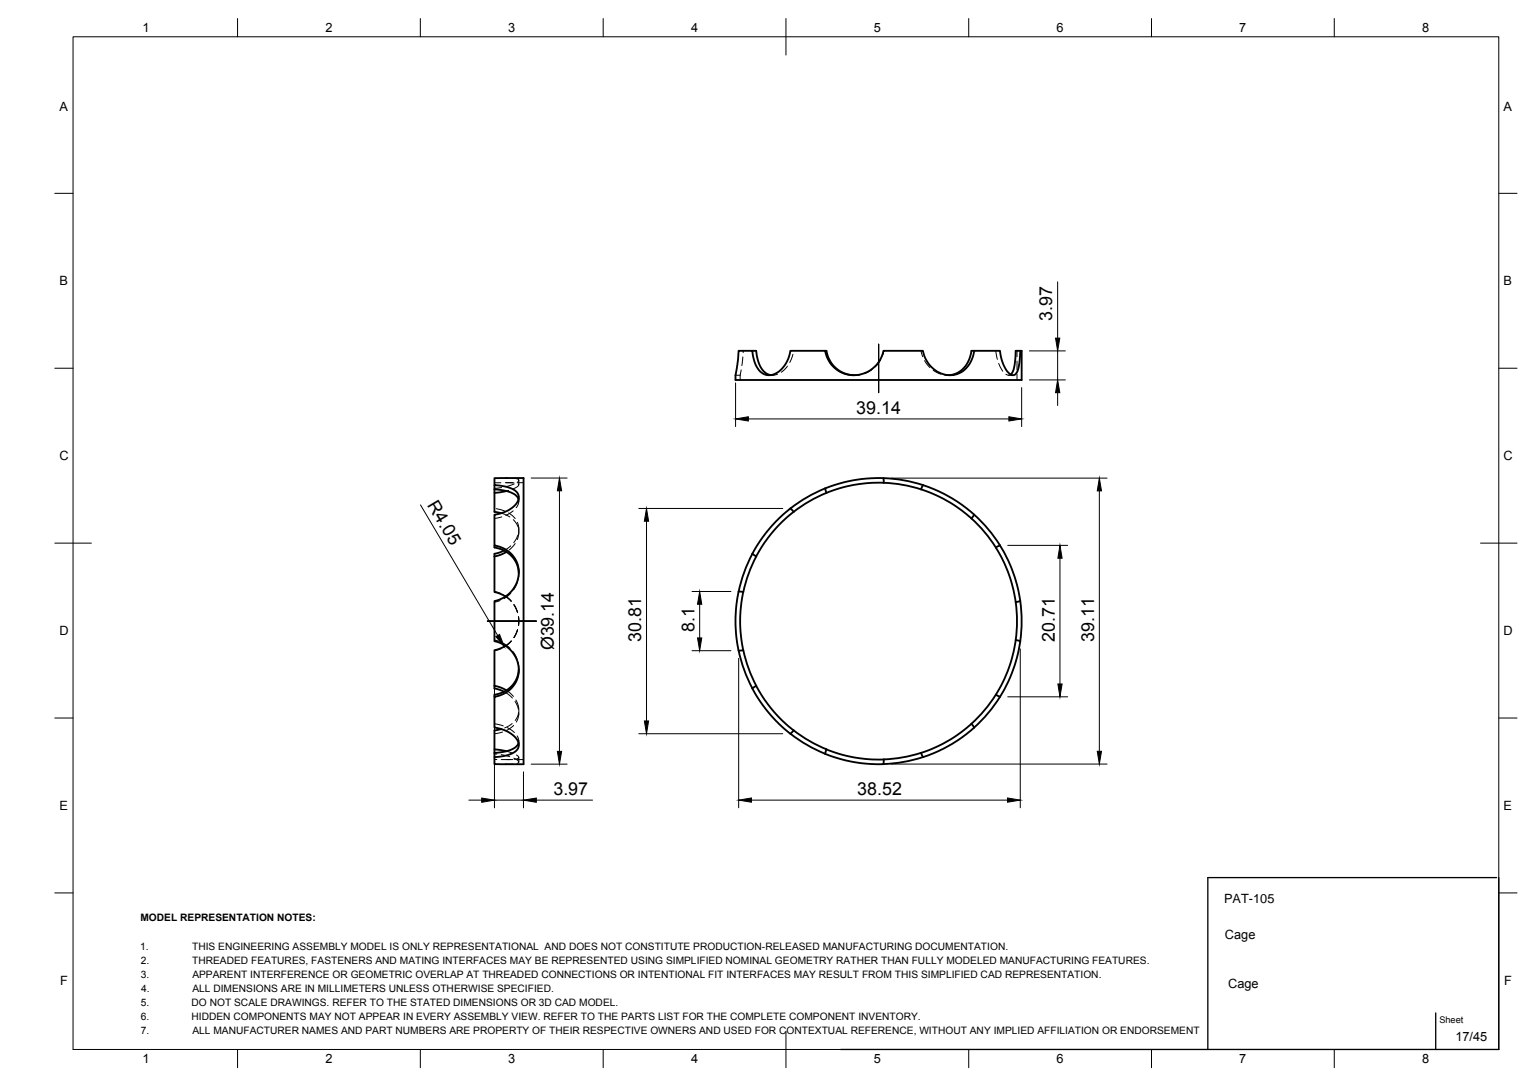
ISO-10303-21;
HEADER;
/* Generated by software containing ST-Developer
 * from STEP Tools, Inc. (www.steptools.com) 
 */

FILE_DESCRIPTION(
/* description */ ('Torque wrench calibration arm'),
/* implementation_level */ '2;1');

FILE_NAME(
/* name */ 'Cage.step',
/* time_stamp */ '2026-10-28T03:24:52-07:00',
/* author */ (''),
/* organization */ (''),
/* preprocessor_version */ 'ST-DEVELOPER v20.2',
/* originating_system */ 'Autodesk Translation Framework v15.17.0.0',
/* authorisation */ '');

FILE_SCHEMA (('AUTOMOTIVE_DESIGN { 1 0 10303 214 3 1 1 }'));
ENDSEC;

DATA;
#10=MECHANICAL_DESIGN_GEOMETRIC_PRESENTATION_REPRESENTATION('',(#444),#12783);
#245=B_SPLINE_CURVE_WITH_KNOTS('',3,(#10516,#10517,#10518,#10519,#10520,
#10521,#10522,#10523,#10524,#10525,#10526,#10527,#10528,#10529,#10530,#10531,
#10532,#10533,#10534,#10535,#10536,#10537),.UNSPECIFIED.,.F.,.F.,(4,2,2,
2,2,2,2,2,2,2,4),(0.0789043916784349,0.21052649634152,0.31578974451228,
0.421052992683041,0.522171766675512,0.623290540667983,0.724409314660453,
0.825528088652924,0.930791336823684,1.03605458499444,1.16767668965753),
 .UNSPECIFIED.);
#246=B_SPLINE_CURVE_WITH_KNOTS('',3,(#10541,#10542,#10543,#10544,#10545,
#10546,#10547,#10548,#10549,#10550,#10551,#10552,#10553,#10554,#10555,#10556,
#10557,#10558,#10559,#10560,#10561,#10562),.UNSPECIFIED.,.F.,.F.,(4,2,2,
2,2,2,2,2,2,2,4),(0.0774711646211702,0.142095081356994,0.284190162713987,
0.410912155766437,0.514012992401139,0.617113829035841,0.720214665670543,
0.823315502305246,0.950037495357694,1.09213257671469,1.15675649345051),
 .UNSPECIFIED.);
#247=B_SPLINE_CURVE_WITH_KNOTS('',3,(#10568,#10569,#10570,#10571,#10572,
#10573,#10574,#10575,#10576,#10577,#10578,#10579,#10580,#10581,#10582,#10583,
#10584,#10585,#10586,#10587,#10588,#10589),.UNSPECIFIED.,.F.,.F.,(4,2,2,
2,2,2,2,2,2,2,4),(0.0774711646211703,0.142095081356994,0.284190162713988,
0.410912155766436,0.514012992401139,0.617113829035841,0.720214665670544,
0.823315502305246,0.950037495357695,1.09213257671469,1.15675649345051),
 .UNSPECIFIED.);
#248=B_SPLINE_CURVE_WITH_KNOTS('',3,(#10593,#10594,#10595,#10596,#10597,
#10598,#10599,#10600,#10601,#10602,#10603,#10604,#10605,#10606,#10607,#10608,
#10609,#10610,#10611,#10612,#10613,#10614),.UNSPECIFIED.,.F.,.F.,(4,2,2,
2,2,2,2,2,2,2,4),(0.0774711646211702,0.142095081356994,0.284190162713988,
0.410912155766436,0.514012992401139,0.617113829035841,0.720214665670544,
0.823315502305246,0.950037495357695,1.09213257671469,1.15675649345051),
 .UNSPECIFIED.);
#249=B_SPLINE_CURVE_WITH_KNOTS('',3,(#10618,#10619,#10620,#10621,#10622,
#10623,#10624,#10625,#10626,#10627,#10628,#10629,#10630,#10631,#10632,#10633,
#10634,#10635,#10636,#10637,#10638,#10639),.UNSPECIFIED.,.F.,.F.,(4,2,2,
2,2,2,2,2,2,2,4),(0.0774711646211702,0.142095081356994,0.284190162713988,
0.410912155766436,0.514012992401139,0.617113829035842,0.720214665670544,
0.823315502305246,0.950037495357696,1.09213257671469,1.15675649345051),
 .UNSPECIFIED.);
#250=B_SPLINE_CURVE_WITH_KNOTS('',3,(#10648,#10649,#10650,#10651,#10652,
#10653,#10654,#10655,#10656,#10657,#10658,#10659,#10660,#10661,#10662,#10663,
#10664,#10665,#10666,#10667,#10668,#10669),.UNSPECIFIED.,.F.,.F.,(4,2,2,
2,2,2,2,2,2,2,4),(0.0774711646211702,0.142095081356994,0.284190162713987,
0.410912155766436,0.514012992401139,0.617113829035841,0.720214665670543,
0.823315502305246,0.950037495357695,1.09213257671469,1.15675649345051),
 .UNSPECIFIED.);
#251=B_SPLINE_CURVE_WITH_KNOTS('',3,(#10673,#10674,#10675,#10676,#10677,
#10678,#10679,#10680,#10681,#10682,#10683,#10684,#10685,#10686,#10687,#10688,
#10689,#10690,#10691,#10692,#10693,#10694),.UNSPECIFIED.,.F.,.F.,(4,2,2,
2,2,2,2,2,2,2,4),(0.0774711646211702,0.142095081356994,0.284190162713987,
0.410912155766436,0.514012992401139,0.617113829035841,0.720214665670543,
0.823315502305246,0.950037495357695,1.09213257671469,1.15675649345051),
 .UNSPECIFIED.);
#252=B_SPLINE_CURVE_WITH_KNOTS('',3,(#10698,#10699,#10700,#10701,#10702,
#10703,#10704,#10705,#10706,#10707,#10708,#10709,#10710,#10711,#10712,#10713,
#10714,#10715,#10716,#10717,#10718,#10719),.UNSPECIFIED.,.F.,.F.,(4,2,2,
2,2,2,2,2,2,2,4),(0.0774711646211703,0.142095081356994,0.284190162713988,
0.410912155766437,0.514012992401139,0.617113829035841,0.720214665670544,
0.823315502305247,0.950037495357696,1.09213257671469,1.15675649345051),
 .UNSPECIFIED.);
#253=B_SPLINE_CURVE_WITH_KNOTS('',3,(#10723,#10724,#10725,#10726,#10727,
#10728,#10729,#10730,#10731,#10732,#10733,#10734,#10735,#10736,#10737,#10738,
#10739,#10740,#10741,#10742,#10743,#10744),.UNSPECIFIED.,.F.,.F.,(4,2,2,
2,2,2,2,2,2,2,4),(0.0774711646211703,0.142095081356994,0.284190162713987,
0.410912155766436,0.514012992401139,0.617113829035841,0.720214665670543,
0.823315502305245,0.950037495357694,1.09213257671469,1.15675649345051),
 .UNSPECIFIED.);
#254=B_SPLINE_CURVE_WITH_KNOTS('',3,(#10748,#10749,#10750,#10751,#10752,
#10753,#10754,#10755,#10756,#10757,#10758,#10759,#10760,#10761,#10762,#10763,
#10764,#10765,#10766,#10767,#10768,#10769),.UNSPECIFIED.,.F.,.F.,(4,2,2,
2,2,2,2,2,2,2,4),(0.0774711646211703,0.142095081356994,0.284190162713988,
0.410912155766437,0.514012992401139,0.617113829035841,0.720214665670544,
0.823315502305246,0.950037495357695,1.09213257671469,1.15675649345051),
 .UNSPECIFIED.);
#255=B_SPLINE_CURVE_WITH_KNOTS('',3,(#10777,#10778,#10779,#10780,#10781,
#10782,#10783,#10784,#10785,#10786,#10787,#10788,#10789,#10790,#10791,#10792,
#10793,#10794,#10795,#10796,#10797,#10798),.UNSPECIFIED.,.F.,.F.,(4,2,2,
2,2,2,2,2,2,2,4),(0.0789043916784349,0.21052649634152,0.315789744512281,
0.421052992683041,0.522171766675512,0.623290540667983,0.724409314660453,
0.825528088652924,0.930791336823684,1.03605458499444,1.16767668965753),
 .UNSPECIFIED.);
#256=B_SPLINE_CURVE_WITH_KNOTS('',3,(#10806,#10807,#10808,#10809,#10810,
#10811,#10812,#10813,#10814,#10815,#10816,#10817,#10818,#10819,#10820,#10821,
#10822,#10823,#10824,#10825,#10826,#10827),.UNSPECIFIED.,.F.,.F.,(4,2,2,
2,2,2,2,2,2,2,4),(0.0789043916784348,0.210526496341521,0.315789744512281,
0.421052992683042,0.522171766675513,0.623290540667983,0.724409314660454,
0.825528088652925,0.930791336823685,1.03605458499444,1.16767668965753),
 .UNSPECIFIED.);
#257=B_SPLINE_CURVE_WITH_KNOTS('',3,(#10835,#10836,#10837,#10838,#10839,
#10840,#10841,#10842,#10843,#10844,#10845,#10846,#10847,#10848,#10849,#10850,
#10851,#10852,#10853,#10854,#10855,#10856),.UNSPECIFIED.,.F.,.F.,(4,2,2,
2,2,2,2,2,2,2,4),(0.0789043916784349,0.21052649634152,0.31578974451228,
0.421052992683041,0.522171766675511,0.623290540667982,0.724409314660453,
0.825528088652924,0.930791336823685,1.03605458499444,1.16767668965753),
 .UNSPECIFIED.);
#258=B_SPLINE_CURVE_WITH_KNOTS('',3,(#10866,#10867,#10868,#10869,#10870,
#10871,#10872,#10873,#10874,#10875,#10876,#10877,#10878,#10879,#10880,#10881,
#10882,#10883,#10884,#10885,#10886,#10887),.UNSPECIFIED.,.F.,.F.,(4,2,2,
2,2,2,2,2,2,2,4),(0.0789043916784348,0.21052649634152,0.315789744512281,
0.421052992683041,0.522171766675511,0.623290540667982,0.724409314660453,
0.825528088652924,0.930791336823684,1.03605458499444,1.16767668965753),
 .UNSPECIFIED.);
#259=B_SPLINE_CURVE_WITH_KNOTS('',3,(#10895,#10896,#10897,#10898,#10899,
#10900,#10901,#10902,#10903,#10904,#10905,#10906,#10907,#10908,#10909,#10910,
#10911,#10912,#10913,#10914,#10915,#10916),.UNSPECIFIED.,.F.,.F.,(4,2,2,
2,2,2,2,2,2,2,4),(0.0789043916784348,0.21052649634152,0.31578974451228,
0.42105299268304,0.522171766675511,0.623290540667982,0.724409314660453,
0.825528088652924,0.930791336823684,1.03605458499444,1.16767668965753),
 .UNSPECIFIED.);
#260=B_SPLINE_CURVE_WITH_KNOTS('',3,(#10924,#10925,#10926,#10927,#10928,
#10929,#10930,#10931,#10932,#10933,#10934,#10935,#10936,#10937,#10938,#10939,
#10940,#10941,#10942,#10943,#10944,#10945),.UNSPECIFIED.,.F.,.F.,(4,2,2,
2,2,2,2,2,2,2,4),(0.0789043916784348,0.21052649634152,0.315789744512281,
0.421052992683041,0.522171766675512,0.623290540667982,0.724409314660453,
0.825528088652924,0.930791336823684,1.03605458499444,1.16767668965753),
 .UNSPECIFIED.);
#261=B_SPLINE_CURVE_WITH_KNOTS('',3,(#10953,#10954,#10955,#10956,#10957,
#10958,#10959,#10960,#10961,#10962,#10963,#10964,#10965,#10966,#10967,#10968,
#10969,#10970,#10971,#10972,#10973,#10974),.UNSPECIFIED.,.F.,.F.,(4,2,2,
2,2,2,2,2,2,2,4),(0.0789043916784349,0.21052649634152,0.31578974451228,
0.42105299268304,0.522171766675511,0.623290540667982,0.724409314660453,
0.825528088652924,0.930791336823684,1.03605458499444,1.16767668965753),
 .UNSPECIFIED.);
#262=B_SPLINE_CURVE_WITH_KNOTS('',3,(#10983,#10984,#10985,#10986,#10987,
#10988,#10989,#10990,#10991,#10992,#10993,#10994,#10995,#10996,#10997,#10998,
#10999,#11000,#11001,#11002,#11003,#11004),.UNSPECIFIED.,.F.,.F.,(4,2,2,
2,2,2,2,2,2,2,4),(0.0789043916784348,0.21052649634152,0.31578974451228,
0.42105299268304,0.522171766675511,0.623290540667982,0.724409314660453,
0.825528088652924,0.930791336823684,1.03605458499444,1.16767668965753),
 .UNSPECIFIED.);
#302=SPHERICAL_SURFACE('',#7218,0.412776);
#303=SPHERICAL_SURFACE('',#7236,0.412776);
#304=SPHERICAL_SURFACE('',#7241,0.412776);
#305=SPHERICAL_SURFACE('',#7246,0.412776);
#306=SPHERICAL_SURFACE('',#7252,0.412776);
#307=SPHERICAL_SURFACE('',#7257,0.412776);
#308=SPHERICAL_SURFACE('',#7262,0.412776);
#309=SPHERICAL_SURFACE('',#7267,0.412776);
#310=SPHERICAL_SURFACE('',#7275,0.412776);
#362=SHAPE_REPRESENTATION_RELATIONSHIP('SRR','None',#12944,#399);
#399=ADVANCED_BREP_SHAPE_REPRESENTATION('',(#498),#12753);
#444=STYLED_ITEM('',(#13212),#498);
#498=MANIFOLD_SOLID_BREP('Continuous crown cage',#6513);
#587=FACE_BOUND('',#1471,.T.);
#714=PLANE('',#7233);
#715=PLANE('',#7238);
#716=PLANE('',#7243);
#717=PLANE('',#7248);
#718=PLANE('',#7254);
#719=PLANE('',#7259);
#720=PLANE('',#7264);
#721=PLANE('',#7273);
#722=PLANE('',#7277);
#723=PLANE('',#7278);
#1000=FACE_OUTER_BOUND('',#1451,.T.);
#1001=FACE_OUTER_BOUND('',#1452,.T.);
#1002=FACE_OUTER_BOUND('',#1453,.T.);
#1003=FACE_OUTER_BOUND('',#1454,.T.);
#1004=FACE_OUTER_BOUND('',#1455,.T.);
#1005=FACE_OUTER_BOUND('',#1456,.T.);
#1006=FACE_OUTER_BOUND('',#1457,.T.);
#1007=FACE_OUTER_BOUND('',#1458,.T.);
#1008=FACE_OUTER_BOUND('',#1459,.T.);
#1009=FACE_OUTER_BOUND('',#1460,.T.);
#1010=FACE_OUTER_BOUND('',#1461,.T.);
#1011=FACE_OUTER_BOUND('',#1462,.T.);
#1012=FACE_OUTER_BOUND('',#1463,.T.);
#1013=FACE_OUTER_BOUND('',#1464,.T.);
#1014=FACE_OUTER_BOUND('',#1465,.T.);
#1015=FACE_OUTER_BOUND('',#1466,.T.);
#1016=FACE_OUTER_BOUND('',#1467,.T.);
#1017=FACE_OUTER_BOUND('',#1468,.T.);
#1018=FACE_OUTER_BOUND('',#1469,.T.);
#1019=FACE_OUTER_BOUND('',#1470,.T.);
#1020=FACE_OUTER_BOUND('',#1472,.T.);
#1451=EDGE_LOOP('',(#4877,#4878,#4879,#4880));
#1452=EDGE_LOOP('',(#4881,#4882,#4883,#4884,#4885,#4886,#4887,#4888,#4889,
#4890,#4891,#4892,#4893,#4894,#4895,#4896,#4897,#4898,#4899,#4900,#4901,
#4902));
#1453=EDGE_LOOP('',(#4903,#4904,#4905,#4906));
#1454=EDGE_LOOP('',(#4907,#4908,#4909,#4910));
#1455=EDGE_LOOP('',(#4911,#4912,#4913,#4914));
#1456=EDGE_LOOP('',(#4915,#4916,#4917,#4918));
#1457=EDGE_LOOP('',(#4919,#4920,#4921,#4922));
#1458=EDGE_LOOP('',(#4923,#4924,#4925,#4926));
#1459=EDGE_LOOP('',(#4927,#4928,#4929,#4930,#4931,#4932));
#1460=EDGE_LOOP('',(#4933,#4934,#4935,#4936));
#1461=EDGE_LOOP('',(#4937,#4938,#4939,#4940));
#1462=EDGE_LOOP('',(#4941,#4942,#4943,#4944));
#1463=EDGE_LOOP('',(#4945,#4946,#4947,#4948));
#1464=EDGE_LOOP('',(#4949,#4950,#4951,#4952));
#1465=EDGE_LOOP('',(#4953,#4954,#4955,#4956));
#1466=EDGE_LOOP('',(#4957,#4958,#4959,#4960));
#1467=EDGE_LOOP('',(#4961,#4962,#4963,#4964,#4965,#4966,#4967,#4968,#4969,
#4970,#4971,#4972,#4973,#4974,#4975,#4976,#4977,#4978,#4979,#4980,#4981,
#4982));
#1468=EDGE_LOOP('',(#4983,#4984,#4985,#4986));
#1469=EDGE_LOOP('',(#4987,#4988,#4989,#4990));
#1470=EDGE_LOOP('',(#4991));
#1471=EDGE_LOOP('',(#4992));
#1472=EDGE_LOOP('',(#4993,#4994,#4995,#4996));
#1930=LINE('',#10643,#2345);
#1931=LINE('',#10979,#2346);
#2345=VECTOR('',#8486,1.956752);
#2346=VECTOR('',#8577,1.893248);
#2735=CIRCLE('',#7219,0.405071403305639);
#2736=CIRCLE('',#7220,0.405071403305639);
#2737=CIRCLE('',#7222,1.956752);
#2738=CIRCLE('',#7223,1.956752);
#2739=CIRCLE('',#7224,1.956752);
#2740=CIRCLE('',#7225,1.956752);
#2741=CIRCLE('',#7226,1.956752);
#2742=CIRCLE('',#7227,1.956752);
#2743=CIRCLE('',#7228,1.956752);
#2744=CIRCLE('',#7229,1.956752);
#2745=CIRCLE('',#7230,1.956752);
#2746=CIRCLE('',#7231,1.956752);
#2747=CIRCLE('',#7232,1.956752);
#2748=CIRCLE('',#7234,1.893248);
#2749=CIRCLE('',#7235,0.405071403305639);
#2750=CIRCLE('',#7237,0.405071403305639);
#2751=CIRCLE('',#7239,1.893248);
#2752=CIRCLE('',#7240,0.405071403305639);
#2753=CIRCLE('',#7242,0.405071403305639);
#2754=CIRCLE('',#7244,1.893248);
#2755=CIRCLE('',#7245,0.405071403305639);
#2756=CIRCLE('',#7247,0.405071403305639);
#2757=CIRCLE('',#7249,1.893248);
#2758=CIRCLE('',#7250,1.893248);
#2759=CIRCLE('',#7251,0.405071403305639);
#2760=CIRCLE('',#7253,0.405071403305639);
#2761=CIRCLE('',#7255,1.893248);
#2762=CIRCLE('',#7256,0.405071403305639);
#2763=CIRCLE('',#7258,0.405071403305639);
#2764=CIRCLE('',#7260,1.893248);
#2765=CIRCLE('',#7261,0.405071403305639);
#2766=CIRCLE('',#7263,0.405071403305639);
#2767=CIRCLE('',#7265,1.893248);
#2768=CIRCLE('',#7266,0.405071403305639);
#2769=CIRCLE('',#7268,0.405071403305639);
#2770=CIRCLE('',#7270,1.893248);
#2771=CIRCLE('',#7271,1.893248);
#2772=CIRCLE('',#7272,1.893248);
#2773=CIRCLE('',#7274,0.405071403305639);
#2774=CIRCLE('',#7276,0.405071403305639);
#3157=VERTEX_POINT('',#10514);
#3158=VERTEX_POINT('',#10515);
#3159=VERTEX_POINT('',#10538);
#3160=VERTEX_POINT('',#10540);
#3161=VERTEX_POINT('',#10565);
#3162=VERTEX_POINT('',#10567);
#3163=VERTEX_POINT('',#10590);
#3164=VERTEX_POINT('',#10592);
#3165=VERTEX_POINT('',#10615);
#3166=VERTEX_POINT('',#10617);
#3167=VERTEX_POINT('',#10640);
#3168=VERTEX_POINT('',#10642);
#3169=VERTEX_POINT('',#10645);
#3170=VERTEX_POINT('',#10647);
#3171=VERTEX_POINT('',#10670);
#3172=VERTEX_POINT('',#10672);
#3173=VERTEX_POINT('',#10695);
#3174=VERTEX_POINT('',#10697);
#3175=VERTEX_POINT('',#10720);
#3176=VERTEX_POINT('',#10722);
#3177=VERTEX_POINT('',#10745);
#3178=VERTEX_POINT('',#10747);
#3179=VERTEX_POINT('',#10772);
#3180=VERTEX_POINT('',#10776);
#3181=VERTEX_POINT('',#10801);
#3182=VERTEX_POINT('',#10805);
#3183=VERTEX_POINT('',#10830);
#3184=VERTEX_POINT('',#10834);
#3185=VERTEX_POINT('',#10859);
#3186=VERTEX_POINT('',#10861);
#3187=VERTEX_POINT('',#10865);
#3188=VERTEX_POINT('',#10890);
#3189=VERTEX_POINT('',#10894);
#3190=VERTEX_POINT('',#10919);
#3191=VERTEX_POINT('',#10923);
#3192=VERTEX_POINT('',#10948);
#3193=VERTEX_POINT('',#10952);
#3194=VERTEX_POINT('',#10977);
#3195=VERTEX_POINT('',#10980);
#3196=VERTEX_POINT('',#10982);
#3796=EDGE_CURVE('',#3157,#3158,#245,.T.);
#3797=EDGE_CURVE('',#3159,#3157,#2735,.T.);
#3798=EDGE_CURVE('',#3160,#3159,#246,.T.);
#3799=EDGE_CURVE('',#3158,#3160,#2736,.T.);
#3800=EDGE_CURVE('',#3161,#3159,#2737,.T.);
#3801=EDGE_CURVE('',#3161,#3162,#247,.T.);
#3802=EDGE_CURVE('',#3163,#3162,#2738,.T.);
#3803=EDGE_CURVE('',#3163,#3164,#248,.T.);
#3804=EDGE_CURVE('',#3165,#3164,#2739,.T.);
#3805=EDGE_CURVE('',#3165,#3166,#249,.T.);
#3806=EDGE_CURVE('',#3167,#3166,#2740,.T.);
#3807=EDGE_CURVE('',#3167,#3168,#1930,.T.);
#3808=EDGE_CURVE('',#3168,#3168,#2741,.T.);
#3809=EDGE_CURVE('',#3169,#3167,#2742,.T.);
#3810=EDGE_CURVE('',#3169,#3170,#250,.T.);
#3811=EDGE_CURVE('',#3171,#3170,#2743,.T.);
#3812=EDGE_CURVE('',#3171,#3172,#251,.T.);
#3813=EDGE_CURVE('',#3173,#3172,#2744,.T.);
#3814=EDGE_CURVE('',#3173,#3174,#252,.T.);
#3815=EDGE_CURVE('',#3175,#3174,#2745,.T.);
#3816=EDGE_CURVE('',#3175,#3176,#253,.T.);
#3817=EDGE_CURVE('',#3177,#3176,#2746,.T.);
#3818=EDGE_CURVE('',#3177,#3178,#254,.T.);
#3819=EDGE_CURVE('',#3160,#3178,#2747,.T.);
#3820=EDGE_CURVE('',#3157,#3179,#2748,.T.);
#3821=EDGE_CURVE('',#3179,#3161,#2749,.T.);
#3822=EDGE_CURVE('',#3180,#3179,#255,.T.);
#3823=EDGE_CURVE('',#3162,#3180,#2750,.T.);
#3824=EDGE_CURVE('',#3180,#3181,#2751,.T.);
#3825=EDGE_CURVE('',#3181,#3163,#2752,.T.);
#3826=EDGE_CURVE('',#3182,#3181,#256,.T.);
#3827=EDGE_CURVE('',#3164,#3182,#2753,.T.);
#3828=EDGE_CURVE('',#3182,#3183,#2754,.T.);
#3829=EDGE_CURVE('',#3183,#3165,#2755,.T.);
#3830=EDGE_CURVE('',#3184,#3183,#257,.T.);
#3831=EDGE_CURVE('',#3166,#3184,#2756,.T.);
#3832=EDGE_CURVE('',#3184,#3185,#2757,.T.);
#3833=EDGE_CURVE('',#3185,#3186,#2758,.T.);
#3834=EDGE_CURVE('',#3186,#3169,#2759,.T.);
#3835=EDGE_CURVE('',#3187,#3186,#258,.T.);
#3836=EDGE_CURVE('',#3170,#3187,#2760,.T.);
#3837=EDGE_CURVE('',#3187,#3188,#2761,.T.);
#3838=EDGE_CURVE('',#3188,#3171,#2762,.T.);
#3839=EDGE_CURVE('',#3189,#3188,#259,.T.);
#3840=EDGE_CURVE('',#3172,#3189,#2763,.T.);
#3841=EDGE_CURVE('',#3189,#3190,#2764,.T.);
#3842=EDGE_CURVE('',#3190,#3173,#2765,.T.);
#3843=EDGE_CURVE('',#3191,#3190,#260,.T.);
#3844=EDGE_CURVE('',#3174,#3191,#2766,.T.);
#3845=EDGE_CURVE('',#3191,#3192,#2767,.T.);
#3846=EDGE_CURVE('',#3192,#3175,#2768,.T.);
#3847=EDGE_CURVE('',#3193,#3192,#261,.T.);
#3848=EDGE_CURVE('',#3176,#3193,#2769,.T.);
#3849=EDGE_CURVE('',#3194,#3194,#2770,.T.);
#3850=EDGE_CURVE('',#3194,#3185,#1931,.T.);
#3851=EDGE_CURVE('',#3195,#3158,#2771,.T.);
#3852=EDGE_CURVE('',#3195,#3196,#262,.T.);
#3853=EDGE_CURVE('',#3193,#3196,#2772,.T.);
#3854=EDGE_CURVE('',#3178,#3195,#2773,.T.);
#3855=EDGE_CURVE('',#3196,#3177,#2774,.T.);
#4877=ORIENTED_EDGE('',*,*,#3796,.F.);
#4878=ORIENTED_EDGE('',*,*,#3797,.F.);
#4879=ORIENTED_EDGE('',*,*,#3798,.F.);
#4880=ORIENTED_EDGE('',*,*,#3799,.F.);
#4881=ORIENTED_EDGE('',*,*,#3798,.T.);
#4882=ORIENTED_EDGE('',*,*,#3800,.F.);
#4883=ORIENTED_EDGE('',*,*,#3801,.T.);
#4884=ORIENTED_EDGE('',*,*,#3802,.F.);
#4885=ORIENTED_EDGE('',*,*,#3803,.T.);
#4886=ORIENTED_EDGE('',*,*,#3804,.F.);
#4887=ORIENTED_EDGE('',*,*,#3805,.T.);
#4888=ORIENTED_EDGE('',*,*,#3806,.F.);
#4889=ORIENTED_EDGE('',*,*,#3807,.T.);
#4890=ORIENTED_EDGE('',*,*,#3808,.F.);
#4891=ORIENTED_EDGE('',*,*,#3807,.F.);
#4892=ORIENTED_EDGE('',*,*,#3809,.F.);
#4893=ORIENTED_EDGE('',*,*,#3810,.T.);
#4894=ORIENTED_EDGE('',*,*,#3811,.F.);
#4895=ORIENTED_EDGE('',*,*,#3812,.T.);
#4896=ORIENTED_EDGE('',*,*,#3813,.F.);
#4897=ORIENTED_EDGE('',*,*,#3814,.T.);
#4898=ORIENTED_EDGE('',*,*,#3815,.F.);
#4899=ORIENTED_EDGE('',*,*,#3816,.T.);
#4900=ORIENTED_EDGE('',*,*,#3817,.F.);
#4901=ORIENTED_EDGE('',*,*,#3818,.T.);
#4902=ORIENTED_EDGE('',*,*,#3819,.F.);
#4903=ORIENTED_EDGE('',*,*,#3797,.T.);
#4904=ORIENTED_EDGE('',*,*,#3820,.T.);
#4905=ORIENTED_EDGE('',*,*,#3821,.T.);
#4906=ORIENTED_EDGE('',*,*,#3800,.T.);
#4907=ORIENTED_EDGE('',*,*,#3822,.F.);
#4908=ORIENTED_EDGE('',*,*,#3823,.F.);
#4909=ORIENTED_EDGE('',*,*,#3801,.F.);
#4910=ORIENTED_EDGE('',*,*,#3821,.F.);
#4911=ORIENTED_EDGE('',*,*,#3823,.T.);
#4912=ORIENTED_EDGE('',*,*,#3824,.T.);
#4913=ORIENTED_EDGE('',*,*,#3825,.T.);
#4914=ORIENTED_EDGE('',*,*,#3802,.T.);
#4915=ORIENTED_EDGE('',*,*,#3826,.F.);
#4916=ORIENTED_EDGE('',*,*,#3827,.F.);
#4917=ORIENTED_EDGE('',*,*,#3803,.F.);
#4918=ORIENTED_EDGE('',*,*,#3825,.F.);
#4919=ORIENTED_EDGE('',*,*,#3827,.T.);
#4920=ORIENTED_EDGE('',*,*,#3828,.T.);
#4921=ORIENTED_EDGE('',*,*,#3829,.T.);
#4922=ORIENTED_EDGE('',*,*,#3804,.T.);
#4923=ORIENTED_EDGE('',*,*,#3830,.F.);
#4924=ORIENTED_EDGE('',*,*,#3831,.F.);
#4925=ORIENTED_EDGE('',*,*,#3805,.F.);
#4926=ORIENTED_EDGE('',*,*,#3829,.F.);
#4927=ORIENTED_EDGE('',*,*,#3831,.T.);
#4928=ORIENTED_EDGE('',*,*,#3832,.T.);
#4929=ORIENTED_EDGE('',*,*,#3833,.T.);
#4930=ORIENTED_EDGE('',*,*,#3834,.T.);
#4931=ORIENTED_EDGE('',*,*,#3809,.T.);
#4932=ORIENTED_EDGE('',*,*,#3806,.T.);
#4933=ORIENTED_EDGE('',*,*,#3835,.F.);
#4934=ORIENTED_EDGE('',*,*,#3836,.F.);
#4935=ORIENTED_EDGE('',*,*,#3810,.F.);
#4936=ORIENTED_EDGE('',*,*,#3834,.F.);
#4937=ORIENTED_EDGE('',*,*,#3836,.T.);
#4938=ORIENTED_EDGE('',*,*,#3837,.T.);
#4939=ORIENTED_EDGE('',*,*,#3838,.T.);
#4940=ORIENTED_EDGE('',*,*,#3811,.T.);
#4941=ORIENTED_EDGE('',*,*,#3839,.F.);
#4942=ORIENTED_EDGE('',*,*,#3840,.F.);
#4943=ORIENTED_EDGE('',*,*,#3812,.F.);
#4944=ORIENTED_EDGE('',*,*,#3838,.F.);
#4945=ORIENTED_EDGE('',*,*,#3840,.T.);
#4946=ORIENTED_EDGE('',*,*,#3841,.T.);
#4947=ORIENTED_EDGE('',*,*,#3842,.T.);
#4948=ORIENTED_EDGE('',*,*,#3813,.T.);
#4949=ORIENTED_EDGE('',*,*,#3843,.F.);
#4950=ORIENTED_EDGE('',*,*,#3844,.F.);
#4951=ORIENTED_EDGE('',*,*,#3814,.F.);
#4952=ORIENTED_EDGE('',*,*,#3842,.F.);
#4953=ORIENTED_EDGE('',*,*,#3844,.T.);
#4954=ORIENTED_EDGE('',*,*,#3845,.T.);
#4955=ORIENTED_EDGE('',*,*,#3846,.T.);
#4956=ORIENTED_EDGE('',*,*,#3815,.T.);
#4957=ORIENTED_EDGE('',*,*,#3816,.F.);
#4958=ORIENTED_EDGE('',*,*,#3846,.F.);
#4959=ORIENTED_EDGE('',*,*,#3847,.F.);
#4960=ORIENTED_EDGE('',*,*,#3848,.F.);
#4961=ORIENTED_EDGE('',*,*,#3849,.F.);
#4962=ORIENTED_EDGE('',*,*,#3850,.T.);
#4963=ORIENTED_EDGE('',*,*,#3832,.F.);
#4964=ORIENTED_EDGE('',*,*,#3830,.T.);
#4965=ORIENTED_EDGE('',*,*,#3828,.F.);
#4966=ORIENTED_EDGE('',*,*,#3826,.T.);
#4967=ORIENTED_EDGE('',*,*,#3824,.F.);
#4968=ORIENTED_EDGE('',*,*,#3822,.T.);
#4969=ORIENTED_EDGE('',*,*,#3820,.F.);
#4970=ORIENTED_EDGE('',*,*,#3796,.T.);
#4971=ORIENTED_EDGE('',*,*,#3851,.F.);
#4972=ORIENTED_EDGE('',*,*,#3852,.T.);
#4973=ORIENTED_EDGE('',*,*,#3853,.F.);
#4974=ORIENTED_EDGE('',*,*,#3847,.T.);
#4975=ORIENTED_EDGE('',*,*,#3845,.F.);
#4976=ORIENTED_EDGE('',*,*,#3843,.T.);
#4977=ORIENTED_EDGE('',*,*,#3841,.F.);
#4978=ORIENTED_EDGE('',*,*,#3839,.T.);
#4979=ORIENTED_EDGE('',*,*,#3837,.F.);
#4980=ORIENTED_EDGE('',*,*,#3835,.T.);
#4981=ORIENTED_EDGE('',*,*,#3833,.F.);
#4982=ORIENTED_EDGE('',*,*,#3850,.F.);
#4983=ORIENTED_EDGE('',*,*,#3799,.T.);
#4984=ORIENTED_EDGE('',*,*,#3819,.T.);
#4985=ORIENTED_EDGE('',*,*,#3854,.T.);
#4986=ORIENTED_EDGE('',*,*,#3851,.T.);
#4987=ORIENTED_EDGE('',*,*,#3818,.F.);
#4988=ORIENTED_EDGE('',*,*,#3855,.F.);
#4989=ORIENTED_EDGE('',*,*,#3852,.F.);
#4990=ORIENTED_EDGE('',*,*,#3854,.F.);
#4991=ORIENTED_EDGE('',*,*,#3808,.T.);
#4992=ORIENTED_EDGE('',*,*,#3849,.T.);
#4993=ORIENTED_EDGE('',*,*,#3848,.T.);
#4994=ORIENTED_EDGE('',*,*,#3853,.T.);
#4995=ORIENTED_EDGE('',*,*,#3855,.T.);
#4996=ORIENTED_EDGE('',*,*,#3817,.T.);
#6035=CYLINDRICAL_SURFACE('',#7221,1.956752);
#6036=CYLINDRICAL_SURFACE('',#7269,1.893248);
#6225=ADVANCED_FACE('',(#1000),#302,.F.);
#6226=ADVANCED_FACE('',(#1001),#6035,.T.);
#6227=ADVANCED_FACE('',(#1002),#714,.T.);
#6228=ADVANCED_FACE('',(#1003),#303,.F.);
#6229=ADVANCED_FACE('',(#1004),#715,.T.);
#6230=ADVANCED_FACE('',(#1005),#304,.F.);
#6231=ADVANCED_FACE('',(#1006),#716,.T.);
#6232=ADVANCED_FACE('',(#1007),#305,.F.);
#6233=ADVANCED_FACE('',(#1008),#717,.T.);
#6234=ADVANCED_FACE('',(#1009),#306,.F.);
#6235=ADVANCED_FACE('',(#1010),#718,.T.);
#6236=ADVANCED_FACE('',(#1011),#307,.F.);
#6237=ADVANCED_FACE('',(#1012),#719,.T.);
#6238=ADVANCED_FACE('',(#1013),#308,.F.);
#6239=ADVANCED_FACE('',(#1014),#720,.T.);
#6240=ADVANCED_FACE('',(#1015),#309,.F.);
#6241=ADVANCED_FACE('',(#1016),#6036,.F.);
#6242=ADVANCED_FACE('',(#1017),#721,.T.);
#6243=ADVANCED_FACE('',(#1018),#310,.F.);
#6244=ADVANCED_FACE('',(#1019,#587),#722,.T.);
#6245=ADVANCED_FACE('',(#1020),#723,.T.);
#6513=CLOSED_SHELL('',(#6225,#6226,#6227,#6228,#6229,#6230,#6231,#6232,
#6233,#6234,#6235,#6236,#6237,#6238,#6239,#6240,#6241,#6242,#6243,#6244,
#6245));
#7217=AXIS2_PLACEMENT_3D('',#10512,#8468,#8469);
#7218=AXIS2_PLACEMENT_3D('',#10513,#8470,#8471);
#7219=AXIS2_PLACEMENT_3D('',#10539,#8472,#8473);
#7220=AXIS2_PLACEMENT_3D('',#10563,#8474,#8475);
#7221=AXIS2_PLACEMENT_3D('',#10564,#8476,#8477);
#7222=AXIS2_PLACEMENT_3D('',#10566,#8478,#8479);
#7223=AXIS2_PLACEMENT_3D('',#10591,#8480,#8481);
#7224=AXIS2_PLACEMENT_3D('',#10616,#8482,#8483);
#7225=AXIS2_PLACEMENT_3D('',#10641,#8484,#8485);
#7226=AXIS2_PLACEMENT_3D('',#10644,#8487,#8488);
#7227=AXIS2_PLACEMENT_3D('',#10646,#8489,#8490);
#7228=AXIS2_PLACEMENT_3D('',#10671,#8491,#8492);
#7229=AXIS2_PLACEMENT_3D('',#10696,#8493,#8494);
#7230=AXIS2_PLACEMENT_3D('',#10721,#8495,#8496);
#7231=AXIS2_PLACEMENT_3D('',#10746,#8497,#8498);
#7232=AXIS2_PLACEMENT_3D('',#10770,#8499,#8500);
#7233=AXIS2_PLACEMENT_3D('',#10771,#8501,#8502);
#7234=AXIS2_PLACEMENT_3D('',#10773,#8503,#8504);
#7235=AXIS2_PLACEMENT_3D('',#10774,#8505,#8506);
#7236=AXIS2_PLACEMENT_3D('',#10775,#8507,#8508);
#7237=AXIS2_PLACEMENT_3D('',#10799,#8509,#8510);
#7238=AXIS2_PLACEMENT_3D('',#10800,#8511,#8512);
#7239=AXIS2_PLACEMENT_3D('',#10802,#8513,#8514);
#7240=AXIS2_PLACEMENT_3D('',#10803,#8515,#8516);
#7241=AXIS2_PLACEMENT_3D('',#10804,#8517,#8518);
#7242=AXIS2_PLACEMENT_3D('',#10828,#8519,#8520);
#7243=AXIS2_PLACEMENT_3D('',#10829,#8521,#8522);
#7244=AXIS2_PLACEMENT_3D('',#10831,#8523,#8524);
#7245=AXIS2_PLACEMENT_3D('',#10832,#8525,#8526);
#7246=AXIS2_PLACEMENT_3D('',#10833,#8527,#8528);
#7247=AXIS2_PLACEMENT_3D('',#10857,#8529,#8530);
#7248=AXIS2_PLACEMENT_3D('',#10858,#8531,#8532);
#7249=AXIS2_PLACEMENT_3D('',#10860,#8533,#8534);
#7250=AXIS2_PLACEMENT_3D('',#10862,#8535,#8536);
#7251=AXIS2_PLACEMENT_3D('',#10863,#8537,#8538);
#7252=AXIS2_PLACEMENT_3D('',#10864,#8539,#8540);
#7253=AXIS2_PLACEMENT_3D('',#10888,#8541,#8542);
#7254=AXIS2_PLACEMENT_3D('',#10889,#8543,#8544);
#7255=AXIS2_PLACEMENT_3D('',#10891,#8545,#8546);
#7256=AXIS2_PLACEMENT_3D('',#10892,#8547,#8548);
#7257=AXIS2_PLACEMENT_3D('',#10893,#8549,#8550);
#7258=AXIS2_PLACEMENT_3D('',#10917,#8551,#8552);
#7259=AXIS2_PLACEMENT_3D('',#10918,#8553,#8554);
#7260=AXIS2_PLACEMENT_3D('',#10920,#8555,#8556);
#7261=AXIS2_PLACEMENT_3D('',#10921,#8557,#8558);
#7262=AXIS2_PLACEMENT_3D('',#10922,#8559,#8560);
#7263=AXIS2_PLACEMENT_3D('',#10946,#8561,#8562);
#7264=AXIS2_PLACEMENT_3D('',#10947,#8563,#8564);
#7265=AXIS2_PLACEMENT_3D('',#10949,#8565,#8566);
#7266=AXIS2_PLACEMENT_3D('',#10950,#8567,#8568);
#7267=AXIS2_PLACEMENT_3D('',#10951,#8569,#8570);
#7268=AXIS2_PLACEMENT_3D('',#10975,#8571,#8572);
#7269=AXIS2_PLACEMENT_3D('',#10976,#8573,#8574);
#7270=AXIS2_PLACEMENT_3D('',#10978,#8575,#8576);
#7271=AXIS2_PLACEMENT_3D('',#10981,#8578,#8579);
#7272=AXIS2_PLACEMENT_3D('',#11005,#8580,#8581);
#7273=AXIS2_PLACEMENT_3D('',#11006,#8582,#8583);
#7274=AXIS2_PLACEMENT_3D('',#11007,#8584,#8585);
#7275=AXIS2_PLACEMENT_3D('',#11008,#8586,#8587);
#7276=AXIS2_PLACEMENT_3D('',#11009,#8588,#8589);
#7277=AXIS2_PLACEMENT_3D('',#11010,#8590,#8591);
#7278=AXIS2_PLACEMENT_3D('',#11011,#8592,#8593);
#8468=DIRECTION('axis',(0.,0.,1.));
#8469=DIRECTION('refdir',(1.,0.,0.));
#8470=DIRECTION('center_axis',(0.,0.,1.));
#8471=DIRECTION('ref_axis',(1.,0.,0.));
#8472=DIRECTION('center_axis',(0.,-1.,0.));
#8473=DIRECTION('ref_axis',(0.,0.,-1.));
#8474=DIRECTION('center_axis',(0.,-1.,0.));
#8475=DIRECTION('ref_axis',(0.,0.,-1.));
#8476=DIRECTION('center_axis',(0.,1.,0.));
#8477=DIRECTION('ref_axis',(1.,0.,0.));
#8478=DIRECTION('center_axis',(0.,1.,0.));
#8479=DIRECTION('ref_axis',(1.,0.,0.));
#8480=DIRECTION('center_axis',(0.,1.,0.));
#8481=DIRECTION('ref_axis',(1.,0.,0.));
#8482=DIRECTION('center_axis',(0.,1.,0.));
#8483=DIRECTION('ref_axis',(1.,0.,0.));
#8484=DIRECTION('center_axis',(0.,1.,0.));
#8485=DIRECTION('ref_axis',(1.,0.,0.));
#8486=DIRECTION('',(0.,-1.,0.));
#8487=DIRECTION('center_axis',(0.,-1.,0.));
#8488=DIRECTION('ref_axis',(1.,0.,0.));
#8489=DIRECTION('center_axis',(0.,1.,0.));
#8490=DIRECTION('ref_axis',(1.,0.,0.));
#8491=DIRECTION('center_axis',(0.,1.,0.));
#8492=DIRECTION('ref_axis',(1.,0.,0.));
#8493=DIRECTION('center_axis',(0.,1.,0.));
#8494=DIRECTION('ref_axis',(1.,0.,0.));
#8495=DIRECTION('center_axis',(0.,1.,0.));
#8496=DIRECTION('ref_axis',(1.,0.,0.));
#8497=DIRECTION('center_axis',(0.,1.,0.));
#8498=DIRECTION('ref_axis',(1.,0.,0.));
#8499=DIRECTION('center_axis',(0.,1.,0.));
#8500=DIRECTION('ref_axis',(1.,0.,0.));
#8501=DIRECTION('center_axis',(0.,1.,0.));
#8502=DIRECTION('ref_axis',(1.,0.,0.));
#8503=DIRECTION('center_axis',(0.,-1.,0.));
#8504=DIRECTION('ref_axis',(1.,0.,0.));
#8505=DIRECTION('center_axis',(0.,-1.,0.));
#8506=DIRECTION('ref_axis',(0.,0.,-1.));
#8507=DIRECTION('center_axis',(0.,0.,1.));
#8508=DIRECTION('ref_axis',(1.,0.,0.));
#8509=DIRECTION('center_axis',(0.,-1.,0.));
#8510=DIRECTION('ref_axis',(0.,0.,-1.));
#8511=DIRECTION('center_axis',(0.,1.,0.));
#8512=DIRECTION('ref_axis',(1.,0.,0.));
#8513=DIRECTION('center_axis',(0.,-1.,0.));
#8514=DIRECTION('ref_axis',(1.,0.,0.));
#8515=DIRECTION('center_axis',(0.,-1.,0.));
#8516=DIRECTION('ref_axis',(0.,0.,-1.));
#8517=DIRECTION('center_axis',(0.,0.,1.));
#8518=DIRECTION('ref_axis',(1.,0.,0.));
#8519=DIRECTION('center_axis',(0.,-1.,0.));
#8520=DIRECTION('ref_axis',(0.,0.,-1.));
#8521=DIRECTION('center_axis',(0.,1.,0.));
#8522=DIRECTION('ref_axis',(1.,0.,0.));
#8523=DIRECTION('center_axis',(0.,-1.,0.));
#8524=DIRECTION('ref_axis',(1.,0.,0.));
#8525=DIRECTION('center_axis',(0.,-1.,0.));
#8526=DIRECTION('ref_axis',(0.,0.,-1.));
#8527=DIRECTION('center_axis',(0.,0.,1.));
#8528=DIRECTION('ref_axis',(1.,0.,0.));
#8529=DIRECTION('center_axis',(0.,-1.,0.));
#8530=DIRECTION('ref_axis',(0.,0.,-1.));
#8531=DIRECTION('center_axis',(0.,1.,0.));
#8532=DIRECTION('ref_axis',(1.,0.,0.));
#8533=DIRECTION('center_axis',(0.,-1.,0.));
#8534=DIRECTION('ref_axis',(1.,0.,0.));
#8535=DIRECTION('center_axis',(0.,-1.,0.));
#8536=DIRECTION('ref_axis',(1.,0.,0.));
#8537=DIRECTION('center_axis',(0.,-1.,0.));
#8538=DIRECTION('ref_axis',(0.,0.,-1.));
#8539=DIRECTION('center_axis',(0.,0.,1.));
#8540=DIRECTION('ref_axis',(1.,0.,0.));
#8541=DIRECTION('center_axis',(0.,-1.,0.));
#8542=DIRECTION('ref_axis',(0.,0.,-1.));
#8543=DIRECTION('center_axis',(0.,1.,0.));
#8544=DIRECTION('ref_axis',(1.,0.,0.));
#8545=DIRECTION('center_axis',(0.,-1.,0.));
#8546=DIRECTION('ref_axis',(1.,0.,0.));
#8547=DIRECTION('center_axis',(0.,-1.,0.));
#8548=DIRECTION('ref_axis',(0.,0.,-1.));
#8549=DIRECTION('center_axis',(0.,0.,1.));
#8550=DIRECTION('ref_axis',(1.,0.,0.));
#8551=DIRECTION('center_axis',(0.,-1.,0.));
#8552=DIRECTION('ref_axis',(0.,0.,-1.));
#8553=DIRECTION('center_axis',(0.,1.,0.));
#8554=DIRECTION('ref_axis',(1.,0.,0.));
#8555=DIRECTION('center_axis',(0.,-1.,0.));
#8556=DIRECTION('ref_axis',(1.,0.,0.));
#8557=DIRECTION('center_axis',(0.,-1.,0.));
#8558=DIRECTION('ref_axis',(0.,0.,-1.));
#8559=DIRECTION('center_axis',(0.,0.,1.));
#8560=DIRECTION('ref_axis',(1.,0.,0.));
#8561=DIRECTION('center_axis',(0.,-1.,0.));
#8562=DIRECTION('ref_axis',(0.,0.,-1.));
#8563=DIRECTION('center_axis',(0.,1.,0.));
#8564=DIRECTION('ref_axis',(1.,0.,0.));
#8565=DIRECTION('center_axis',(0.,-1.,0.));
#8566=DIRECTION('ref_axis',(1.,0.,0.));
#8567=DIRECTION('center_axis',(0.,-1.,0.));
#8568=DIRECTION('ref_axis',(0.,0.,-1.));
#8569=DIRECTION('center_axis',(0.,0.,1.));
#8570=DIRECTION('ref_axis',(1.,0.,0.));
#8571=DIRECTION('center_axis',(0.,-1.,0.));
#8572=DIRECTION('ref_axis',(0.,0.,-1.));
#8573=DIRECTION('center_axis',(0.,1.,0.));
#8574=DIRECTION('ref_axis',(1.,0.,0.));
#8575=DIRECTION('center_axis',(0.,1.,0.));
#8576=DIRECTION('ref_axis',(1.,0.,0.));
#8577=DIRECTION('',(0.,1.,0.));
#8578=DIRECTION('center_axis',(0.,-1.,0.));
#8579=DIRECTION('ref_axis',(1.,0.,0.));
#8580=DIRECTION('center_axis',(0.,-1.,0.));
#8581=DIRECTION('ref_axis',(1.,0.,0.));
#8582=DIRECTION('center_axis',(0.,1.,0.));
#8583=DIRECTION('ref_axis',(1.,0.,0.));
#8584=DIRECTION('center_axis',(0.,-1.,0.));
#8585=DIRECTION('ref_axis',(0.,0.,-1.));
#8586=DIRECTION('center_axis',(0.,0.,1.));
#8587=DIRECTION('ref_axis',(1.,0.,0.));
#8588=DIRECTION('center_axis',(0.,-1.,0.));
#8589=DIRECTION('ref_axis',(0.,0.,-1.));
#8590=DIRECTION('center_axis',(0.,-1.,0.));
#8591=DIRECTION('ref_axis',(-1.,0.,0.));
#8592=DIRECTION('center_axis',(0.,1.,0.));
#8593=DIRECTION('ref_axis',(1.,0.,0.));
#10512=CARTESIAN_POINT('',(0.,0.,0.));
#10513=CARTESIAN_POINT('Origin',(1.47463555300403,0.,1.23736614864659));
#10514=CARTESIAN_POINT('',(1.16188454446795,-0.07938,1.49479506783723));
#10515=CARTESIAN_POINT('',(1.67384490577674,-0.07938,0.884664467981643));
#10516=CARTESIAN_POINT('Ctrl Pts',(1.16188454446795,-0.07938,1.49479506783723));
#10517=CARTESIAN_POINT('Ctrl Pts',(1.16869700612251,-0.123392992551698,
1.48949983100074));
#10518=CARTESIAN_POINT('Ctrl Pts',(1.18135446441955,-0.166529565724166,
1.47962830891229));
#10519=CARTESIAN_POINT('Ctrl Pts',(1.21282145231718,-0.237213819614884,
1.45388393800011));
#10520=CARTESIAN_POINT('Ctrl Pts',(1.22989120215288,-0.266247928944116,
1.4395843844684));
#10521=CARTESIAN_POINT('Ctrl Pts',(1.26813946847809,-0.317173992396757,
1.40600777299249));
#10522=CARTESIAN_POINT('Ctrl Pts',(1.28931069477441,-0.339063173951852,
1.38671820696899));
#10523=CARTESIAN_POINT('Ctrl Pts',(1.33224261954459,-0.373566122196588,
1.34549913552853));
#10524=CARTESIAN_POINT('Ctrl Pts',(1.35618281536764,-0.388075792674378,
1.32151296077672));
#10525=CARTESIAN_POINT('Ctrl Pts',(1.40439359896051,-0.407069005705619,
1.27016020894803));
#10526=CARTESIAN_POINT('Ctrl Pts',(1.42864614483643,-0.411552957311693,
1.24277684810113));
#10527=CARTESIAN_POINT('Ctrl Pts',(1.4719780748558,-0.411552957311693,1.19113586482651));
#10528=CARTESIAN_POINT('Ctrl Pts',(1.49473401052622,-0.407069005705619,
1.16249669890816));
#10529=CARTESIAN_POINT('Ctrl Pts',(1.53693488395083,-0.388075792674377,
1.10610103367387));
#10530=CARTESIAN_POINT('Ctrl Pts',(1.55639948343386,-0.373566122196588,
1.07835938768384));
#10531=CARTESIAN_POINT('Ctrl Pts',(1.58953729406031,-0.339063173951852,
1.02892207867768));
#10532=CARTESIAN_POINT('Ctrl Pts',(1.60485746336717,-0.317173992396757,
1.00472289289232));
#10533=CARTESIAN_POINT('Ctrl Pts',(1.63128222892223,-0.266247928944116,
0.961225186280959));
#10534=CARTESIAN_POINT('Ctrl Pts',(1.64240040915267,-0.237213819614884,
0.941931672888549));
#10535=CARTESIAN_POINT('Ctrl Pts',(1.66228948011831,-0.166529565724165,
0.906472276148935));
#10536=CARTESIAN_POINT('Ctrl Pts',(1.66981308703787,-0.123392992551698,
0.892292941263125));
#10537=CARTESIAN_POINT('Ctrl Pts',(1.67384490577674,-0.07938,0.884664467981643));
#10538=CARTESIAN_POINT('',(1.20622598189858,-0.07938,1.54074568637942));
#10539=CARTESIAN_POINT('Origin',(1.47463555300403,-0.07938,1.23736614864659));
#10540=CARTESIAN_POINT('',(1.72679724097776,-0.07938,0.920353018170519));
#10541=CARTESIAN_POINT('Ctrl Pts',(1.72679724097776,-0.0793800000000002,
0.920353018170518));
#10542=CARTESIAN_POINT('Ctrl Pts',(1.72470909046691,-0.10165971810728,0.92427087628551));
#10543=CARTESIAN_POINT('Ctrl Pts',(1.72169532435455,-0.123845306465941,
0.929898398578877));
#10544=CARTESIAN_POINT('Ctrl Pts',(1.70911544962889,-0.192537547974292,
0.952957916220029));
#10545=CARTESIAN_POINT('Ctrl Pts',(1.69580594901181,-0.236239311587943,
0.976785804874841));
#10546=CARTESIAN_POINT('Ctrl Pts',(1.66527150643903,-0.303218781300911,
1.02787962443771));
#10547=CARTESIAN_POINT('Ctrl Pts',(1.64438322958071,-0.3351607303803,1.06123747122987));
#10548=CARTESIAN_POINT('Ctrl Pts',(1.60730731395783,-0.3732673312795,1.11639170354769));
#10549=CARTESIAN_POINT('Ctrl Pts',(1.5873911192195,-0.387903357081022,1.1447096804553));
#10550=CARTESIAN_POINT('Ctrl Pts',(1.54427174765086,-0.40704475551587,1.20224605970712));
#10551=CARTESIAN_POINT('Ctrl Pts',(1.52104964294098,-0.411552957311693,
1.23144933316771));
#10552=CARTESIAN_POINT('Ctrl Pts',(1.47686834938291,-0.411552957311693,
1.284102548491));
#10553=CARTESIAN_POINT('Ctrl Pts',(1.45214121543005,-0.40704475551587,1.31204295246889));
#10554=CARTESIAN_POINT('Ctrl Pts',(1.40296654335764,-0.387903357081022,
1.36449833130133));
#10555=CARTESIAN_POINT('Ctrl Pts',(1.37853719107178,-0.3732673312795,1.38902931937536));
#10556=CARTESIAN_POINT('Ctrl Pts',(1.330659040657,-0.3351607303803,1.43511940046341));
#10557=CARTESIAN_POINT('Ctrl Pts',(1.30143518572334,-0.303218781300911,
1.4614828667669));
#10558=CARTESIAN_POINT('Ctrl Pts',(1.25641984639565,-0.236239311587943,
1.50042577120361));
#10559=CARTESIAN_POINT('Ctrl Pts',(1.23526512743829,-0.192537547974292,
1.51767074004259));
#10560=CARTESIAN_POINT('Ctrl Pts',(1.21474040800595,-0.123845306465941,
1.53406374142061));
#10561=CARTESIAN_POINT('Ctrl Pts',(1.20972171541452,-0.10165971810728,1.53800893064485));
#10562=CARTESIAN_POINT('Ctrl Pts',(1.20622598189858,-0.0793800000000002,
1.54074568637942));
#10563=CARTESIAN_POINT('Origin',(1.47463555300403,-0.07938,1.23736614864659));
#10564=CARTESIAN_POINT('Origin',(0.,-0.27783,0.));
#10565=CARTESIAN_POINT('',(0.731211914226578,-0.07938,1.81499518621871));
#10566=CARTESIAN_POINT('Origin',(0.,-0.07938,0.));
#10567=CARTESIAN_POINT('',(-0.0663495263035324,-0.07938,1.95562678695688));
#10568=CARTESIAN_POINT('Ctrl Pts',(0.73121191422658,-0.0793800000000002,
1.81499518621871));
#10569=CARTESIAN_POINT('Ctrl Pts',(0.727093947478514,-0.10165971810728,
1.81665420238109));
#10570=CARTESIAN_POINT('Ctrl Pts',(0.721167967091869,-0.123845306465941,
1.81902792304693));
#10571=CARTESIAN_POINT('Ctrl Pts',(0.696708851738065,-0.192537547974292,
1.82860635079188));
#10572=CARTESIAN_POINT('Ctrl Pts',(0.671196911157359,-0.236239311587943,
1.83830439039938));
#10573=CARTESIAN_POINT('Ctrl Pts',(0.614963696954177,-0.303218781300911,
1.85781736559878));
#10574=CARTESIAN_POINT('Ctrl Pts',(0.577520337936704,-0.3351607303803,1.86994423321609));
#10575=CARTESIAN_POINT('Ctrl Pts',(0.513666081644577,-0.3732673312795,1.88836288721748));
#10576=CARTESIAN_POINT('Ctrl Pts',(0.48020694664961,-0.387903357081022,
1.89725383285802));
#10577=CARTESIAN_POINT('Ctrl Pts',(0.410191919979371,-0.40704475551587,
1.91361265867928));
#10578=CARTESIAN_POINT('Ctrl Pts',(0.373631253366087,-0.411552957311693,
1.92105678285629));
#10579=CARTESIAN_POINT('Ctrl Pts',(0.305941584526154,-0.411552957311693,
1.932992297788));
#10580=CARTESIAN_POINT('Ctrl Pts',(0.269039755480681,-0.40704475551587,
1.9385015936658));
#10581=CARTESIAN_POINT('Ctrl Pts',(0.197652103622503,-0.387903357081022,
1.94707587521355));
#10582=CARTESIAN_POINT('Ctrl Pts',(0.163169918867575,-0.3732673312795,1.95016481734985));
#10583=CARTESIAN_POINT('Ctrl Pts',(0.09686699474267,-0.3351607303803,1.95469638598893));
#10584=CARTESIAN_POINT('Ctrl Pts',(0.0575341135759475,-0.30321878130091,
1.95610724099344));
#10585=CARTESIAN_POINT('Ctrl Pts',(-0.00198165342826295,-0.236239311587942,
1.95700393417042));
#10586=CARTESIAN_POINT('Ctrl Pts',(-0.0292719606304177,-0.192537547974292,
1.95661635548909));
#10587=CARTESIAN_POINT('Ctrl Pts',(-0.0555320260694991,-0.123845306465941,
1.95598108775736));
#10588=CARTESIAN_POINT('Ctrl Pts',(-0.0619124863920986,-0.10165971810728,
1.95577732462505));
#10589=CARTESIAN_POINT('Ctrl Pts',(-0.0663495263035336,-0.0793800000000002,
1.95562678695688));
#10590=CARTESIAN_POINT('',(-0.606515593706441,-0.07938,1.86038093521056));
#10591=CARTESIAN_POINT('Origin',(0.,-0.07938,0.));
#10592=CARTESIAN_POINT('',(-1.30787935375538,-0.07938,1.45544837954646));
#10593=CARTESIAN_POINT('Ctrl Pts',(-0.60651559370644,-0.0793800000000002,
1.86038093521056));
#10594=CARTESIAN_POINT('Ctrl Pts',(-0.610736534284191,-0.10165971810728,
1.85900483732004));
#10595=CARTESIAN_POINT('Ctrl Pts',(-0.616801896862274,-0.123845306465941,
1.85701406607784));
#10596=CARTESIAN_POINT('Ctrl Pts',(-0.64169556093739,-0.192537547974292,
1.84862955113236));
#10597=CARTESIAN_POINT('Ctrl Pts',(-0.667472620950374,-0.236239311587943,
1.8396599211785));
#10598=CARTESIAN_POINT('Ctrl Pts',(-0.723092460895733,-0.303218781300911,
1.81846171405606));
#10599=CARTESIAN_POINT('Ctrl Pts',(-0.759570738251496,-0.3351607303803,
1.80368330636526));
#10600=CARTESIAN_POINT('Ctrl Pts',(-0.820325219032771,-0.3732673312795,
1.77674808914243));
#10601=CARTESIAN_POINT('Ctrl Pts',(-0.851671393163369,-0.387903357081022,
1.76205183123884));
#10602=CARTESIAN_POINT('Ctrl Pts',(-0.915821265825857,-0.40704475551587,
1.72957862721967));
#10603=CARTESIAN_POINT('Ctrl Pts',(-0.948613352107641,-0.411552957311693,
1.71178041367846));
#10604=CARTESIAN_POINT('Ctrl Pts',(-1.00813864789236,-0.411552957311693,
1.67741346813356));
#10605=CARTESIAN_POINT('Ctrl Pts',(-1.03994839610192,-0.40704475551587,
1.65791379514105));
#10606=CARTESIAN_POINT('Ctrl Pts',(-1.10014595205605,-0.387903357081022,
1.61859497777538));
#10607=CARTESIAN_POINT('Ctrl Pts',(-1.12854637180642,-0.3732673312795,1.59879652361863));
#10608=CARTESIAN_POINT('Ctrl Pts',(-1.18225019456848,-0.3351607303803,1.55964920847973));
#10609=CARTESIAN_POINT('Ctrl Pts',(-1.21328780973407,-0.30321878130091,
1.53544729744874));
#10610=CARTESIAN_POINT('Ctrl Pts',(-1.25945591558947,-0.236239311587942,
1.49787820666285));
#10611=CARTESIAN_POINT('Ctrl Pts',(-1.28011237299855,-0.192537547974292,
1.48003943283366));
#10612=CARTESIAN_POINT('Ctrl Pts',(-1.29982040797731,-0.12384530646594,
1.46267314482408));
#10613=CARTESIAN_POINT('Ctrl Pts',(-1.30457714773522,-0.10165971810728,
1.45841577236939));
#10614=CARTESIAN_POINT('Ctrl Pts',(-1.30787935375538,-0.0793800000000002,
1.45544837954646));
#10615=CARTESIAN_POINT('',(-1.66044771467423,-0.07938,1.03527376878636));
#10616=CARTESIAN_POINT('Origin',(0.,-0.07938,0.));
#10617=CARTESIAN_POINT('',(-1.93743789612516,-0.07938,0.274249499839291));
#10618=CARTESIAN_POINT('Ctrl Pts',(-1.66044771467423,-0.0793800000000002,
1.03527376878636));
#10619=CARTESIAN_POINT('Ctrl Pts',(-1.66279660407481,-0.10165971810728,
1.03150644833954));
#10620=CARTESIAN_POINT('Ctrl Pts',(-1.66616329828505,-0.123845306465941,
1.02608268917849));
#10621=CARTESIAN_POINT('Ctrl Pts',(-1.67984348899847,-0.192537547974292,
1.00365843926907));
#10622=CARTESIAN_POINT('Ctrl Pts',(-1.69382429558355,-0.236239311587943,
0.980218129295584));
#10623=CARTESIAN_POINT('Ctrl Pts',(-1.72280562001498,-0.303218781300911,
0.928227616555729));
#10624=CARTESIAN_POINT('Ctrl Pts',(-1.74125022432338,-0.3351607303803,0.893458914759057));
#10625=CARTESIAN_POINT('Ctrl Pts',(-1.7704772328254,-0.3732673312795,0.833773113802161));
#10626=CARTESIAN_POINT('Ctrl Pts',(-1.785043222842,-0.387903357081022,0.802366194758251));
#10627=CARTESIAN_POINT('Ctrl Pts',(-1.81331150313154,-0.407044755515871,
0.736255533958675));
#10628=CARTESIAN_POINT('Ctrl Pts',(-1.82699122746714,-0.411552957311693,
0.701542964620283));
#10629=CARTESIAN_POINT('Ctrl Pts',(-1.850499602749,-0.411552957311693,0.636954234365294));
#10630=CARTESIAN_POINT('Ctrl Pts',(-1.86233313540942,-0.40704475551587,
0.60156970621039));
#10631=CARTESIAN_POINT('Ctrl Pts',(-1.88317349000725,-0.387903357081022,
0.53275550155669));
#10632=CARTESIAN_POINT('Ctrl Pts',(-1.89220327271636,-0.3732673312795,0.499333567842125));
#10633=CARTESIAN_POINT('Ctrl Pts',(-1.9081793785937,-0.3351607303803,0.434824832752687));
#10634=CARTESIAN_POINT('Ctrl Pts',(-1.91639888267751,-0.30321878130091,
0.396334498831876));
#10635=CARTESIAN_POINT('Ctrl Pts',(-1.92761675755301,-0.236239311587942,
0.337878619195771));
#10636=CARTESIAN_POINT('Ctrl Pts',(-1.93197397917636,-0.192537547974292,
0.310935610749289));
#10637=CARTESIAN_POINT('Ctrl Pts',(-1.93590837509782,-0.12384530646594,
0.284964181626328));
#10638=CARTESIAN_POINT('Ctrl Pts',(-1.93681566289304,-0.10165971810728,
0.278645271736243));
#10639=CARTESIAN_POINT('Ctrl Pts',(-1.93743789612516,-0.0793800000000002,
0.27424949983929));
#10640=CARTESIAN_POINT('',(-1.956752,-0.07938,2.39633007352518E-16));
#10641=CARTESIAN_POINT('Origin',(0.,-0.07938,0.));
#10642=CARTESIAN_POINT('',(-1.956752,-0.47628,2.39633007352518E-16));
#10643=CARTESIAN_POINT('',(-1.956752,-0.27783,2.39633007352518E-16));
#10644=CARTESIAN_POINT('Origin',(0.,-0.47628,0.));
#10645=CARTESIAN_POINT('',(-1.93743789612516,-0.07938,-0.274249499839292));
#10646=CARTESIAN_POINT('Origin',(0.,-0.07938,0.));
#10647=CARTESIAN_POINT('',(-1.66044771467423,-0.07938,-1.03527376878636));
#10648=CARTESIAN_POINT('Ctrl Pts',(-1.93743789612516,-0.0793800000000002,
-0.27424949983929));
#10649=CARTESIAN_POINT('Ctrl Pts',(-1.93681566289304,-0.10165971810728,
-0.278645271736244));
#10650=CARTESIAN_POINT('Ctrl Pts',(-1.93590837509782,-0.123845306465941,
-0.284964181626328));
#10651=CARTESIAN_POINT('Ctrl Pts',(-1.93197397917636,-0.192537547974292,
-0.310935610749289));
#10652=CARTESIAN_POINT('Ctrl Pts',(-1.92761675755301,-0.236239311587942,
-0.337878619195772));
#10653=CARTESIAN_POINT('Ctrl Pts',(-1.91639888267751,-0.303218781300911,
-0.396334498831877));
#10654=CARTESIAN_POINT('Ctrl Pts',(-1.9081793785937,-0.3351607303803,-0.434824832752687));
#10655=CARTESIAN_POINT('Ctrl Pts',(-1.89220327271636,-0.3732673312795,-0.499333567842125));
#10656=CARTESIAN_POINT('Ctrl Pts',(-1.88317349000725,-0.387903357081022,
-0.53275550155669));
#10657=CARTESIAN_POINT('Ctrl Pts',(-1.86233313540942,-0.40704475551587,
-0.601569706210391));
#10658=CARTESIAN_POINT('Ctrl Pts',(-1.850499602749,-0.411552957311693,-0.636954234365295));
#10659=CARTESIAN_POINT('Ctrl Pts',(-1.82699122746714,-0.411552957311693,
-0.701542964620284));
#10660=CARTESIAN_POINT('Ctrl Pts',(-1.81331150313154,-0.40704475551587,
-0.736255533958675));
#10661=CARTESIAN_POINT('Ctrl Pts',(-1.785043222842,-0.387903357081022,-0.802366194758251));
#10662=CARTESIAN_POINT('Ctrl Pts',(-1.7704772328254,-0.3732673312795,-0.833773113802161));
#10663=CARTESIAN_POINT('Ctrl Pts',(-1.74125022432338,-0.3351607303803,-0.893458914759057));
#10664=CARTESIAN_POINT('Ctrl Pts',(-1.72280562001498,-0.303218781300911,
-0.92822761655573));
#10665=CARTESIAN_POINT('Ctrl Pts',(-1.69382429558355,-0.236239311587942,
-0.980218129295584));
#10666=CARTESIAN_POINT('Ctrl Pts',(-1.67984348899847,-0.192537547974292,
-1.00365843926907));
#10667=CARTESIAN_POINT('Ctrl Pts',(-1.66616329828505,-0.123845306465941,
-1.02608268917849));
#10668=CARTESIAN_POINT('Ctrl Pts',(-1.66279660407481,-0.10165971810728,
-1.03150644833954));
#10669=CARTESIAN_POINT('Ctrl Pts',(-1.66044771467423,-0.0793800000000001,
-1.03527376878636));
#10670=CARTESIAN_POINT('',(-1.30787935375538,-0.07938,-1.45544837954646));
#10671=CARTESIAN_POINT('Origin',(0.,-0.07938,0.));
#10672=CARTESIAN_POINT('',(-0.60651559370644,-0.07938,-1.86038093521056));
#10673=CARTESIAN_POINT('Ctrl Pts',(-1.30787935375538,-0.0793800000000002,
-1.45544837954646));
#10674=CARTESIAN_POINT('Ctrl Pts',(-1.30457714773522,-0.10165971810728,
-1.45841577236939));
#10675=CARTESIAN_POINT('Ctrl Pts',(-1.29982040797731,-0.123845306465941,
-1.46267314482408));
#10676=CARTESIAN_POINT('Ctrl Pts',(-1.28011237299855,-0.192537547974292,
-1.48003943283366));
#10677=CARTESIAN_POINT('Ctrl Pts',(-1.25945591558947,-0.236239311587942,
-1.49787820666285));
#10678=CARTESIAN_POINT('Ctrl Pts',(-1.21328780973407,-0.303218781300911,
-1.53544729744874));
#10679=CARTESIAN_POINT('Ctrl Pts',(-1.18225019456848,-0.3351607303803,-1.55964920847973));
#10680=CARTESIAN_POINT('Ctrl Pts',(-1.12854637180642,-0.3732673312795,-1.59879652361863));
#10681=CARTESIAN_POINT('Ctrl Pts',(-1.10014595205605,-0.387903357081022,
-1.61859497777538));
#10682=CARTESIAN_POINT('Ctrl Pts',(-1.03994839610192,-0.40704475551587,
-1.65791379514105));
#10683=CARTESIAN_POINT('Ctrl Pts',(-1.00813864789236,-0.411552957311693,
-1.67741346813356));
#10684=CARTESIAN_POINT('Ctrl Pts',(-0.948613352107639,-0.411552957311693,
-1.71178041367846));
#10685=CARTESIAN_POINT('Ctrl Pts',(-0.915821265825855,-0.40704475551587,
-1.72957862721967));
#10686=CARTESIAN_POINT('Ctrl Pts',(-0.851671393163367,-0.387903357081022,
-1.76205183123885));
#10687=CARTESIAN_POINT('Ctrl Pts',(-0.820325219032769,-0.3732673312795,
-1.77674808914243));
#10688=CARTESIAN_POINT('Ctrl Pts',(-0.759570738251494,-0.3351607303803,
-1.80368330636526));
#10689=CARTESIAN_POINT('Ctrl Pts',(-0.723092460895731,-0.303218781300911,
-1.81846171405606));
#10690=CARTESIAN_POINT('Ctrl Pts',(-0.667472620950373,-0.236239311587942,
-1.8396599211785));
#10691=CARTESIAN_POINT('Ctrl Pts',(-0.641695560937389,-0.192537547974292,
-1.84862955113236));
#10692=CARTESIAN_POINT('Ctrl Pts',(-0.616801896862272,-0.123845306465941,
-1.85701406607784));
#10693=CARTESIAN_POINT('Ctrl Pts',(-0.610736534284189,-0.10165971810728,
-1.85900483732004));
#10694=CARTESIAN_POINT('Ctrl Pts',(-0.606515593706439,-0.0793800000000002,
-1.86038093521056));
#10695=CARTESIAN_POINT('',(-0.0663495263035315,-0.07938,-1.95562678695688));
#10696=CARTESIAN_POINT('Origin',(0.,-0.07938,0.));
#10697=CARTESIAN_POINT('',(0.731211914226579,-0.07938,-1.81499518621871));
#10698=CARTESIAN_POINT('Ctrl Pts',(-0.0663495263035327,-0.0793800000000002,
-1.95562678695688));
#10699=CARTESIAN_POINT('Ctrl Pts',(-0.0619124863920977,-0.10165971810728,
-1.95577732462505));
#10700=CARTESIAN_POINT('Ctrl Pts',(-0.0555320260694982,-0.123845306465941,
-1.95598108775736));
#10701=CARTESIAN_POINT('Ctrl Pts',(-0.0292719606304167,-0.192537547974292,
-1.95661635548909));
#10702=CARTESIAN_POINT('Ctrl Pts',(-0.00198165342826177,-0.236239311587943,
-1.95700393417042));
#10703=CARTESIAN_POINT('Ctrl Pts',(0.0575341135759488,-0.303218781300911,
-1.95610724099344));
#10704=CARTESIAN_POINT('Ctrl Pts',(0.0968669947426714,-0.3351607303803,
-1.95469638598893));
#10705=CARTESIAN_POINT('Ctrl Pts',(0.163169918867576,-0.3732673312795,-1.95016481734985));
#10706=CARTESIAN_POINT('Ctrl Pts',(0.197652103622504,-0.387903357081022,
-1.94707587521355));
#10707=CARTESIAN_POINT('Ctrl Pts',(0.269039755480682,-0.40704475551587,
-1.9385015936658));
#10708=CARTESIAN_POINT('Ctrl Pts',(0.305941584526155,-0.411552957311693,
-1.93299229778799));
#10709=CARTESIAN_POINT('Ctrl Pts',(0.373631253366089,-0.411552957311693,
-1.92105678285629));
#10710=CARTESIAN_POINT('Ctrl Pts',(0.410191919979372,-0.40704475551587,
-1.91361265867928));
#10711=CARTESIAN_POINT('Ctrl Pts',(0.480206946649611,-0.387903357081022,
-1.89725383285802));
#10712=CARTESIAN_POINT('Ctrl Pts',(0.513666081644578,-0.3732673312795,-1.88836288721748));
#10713=CARTESIAN_POINT('Ctrl Pts',(0.577520337936705,-0.3351607303803,-1.86994423321609));
#10714=CARTESIAN_POINT('Ctrl Pts',(0.614963696954178,-0.30321878130091,
-1.85781736559878));
#10715=CARTESIAN_POINT('Ctrl Pts',(0.67119691115736,-0.236239311587942,
-1.83830439039938));
#10716=CARTESIAN_POINT('Ctrl Pts',(0.696708851738067,-0.192537547974292,
-1.82860635079188));
#10717=CARTESIAN_POINT('Ctrl Pts',(0.721167967091869,-0.123845306465941,
-1.81902792304693));
#10718=CARTESIAN_POINT('Ctrl Pts',(0.727093947478515,-0.10165971810728,
-1.81665420238109));
#10719=CARTESIAN_POINT('Ctrl Pts',(0.73121191422658,-0.0793800000000002,
-1.81499518621871));
#10720=CARTESIAN_POINT('',(1.20622598189858,-0.07938,-1.54074568637942));
#10721=CARTESIAN_POINT('Origin',(0.,-0.07938,0.));
#10722=CARTESIAN_POINT('',(1.72679724097776,-0.07938,-0.920353018170518));
#10723=CARTESIAN_POINT('Ctrl Pts',(1.20622598189858,-0.0793800000000002,
-1.54074568637942));
#10724=CARTESIAN_POINT('Ctrl Pts',(1.20972171541452,-0.10165971810728,-1.53800893064485));
#10725=CARTESIAN_POINT('Ctrl Pts',(1.21474040800596,-0.123845306465941,
-1.53406374142061));
#10726=CARTESIAN_POINT('Ctrl Pts',(1.23526512743829,-0.192537547974292,
-1.51767074004259));
#10727=CARTESIAN_POINT('Ctrl Pts',(1.25641984639565,-0.236239311587942,
-1.50042577120361));
#10728=CARTESIAN_POINT('Ctrl Pts',(1.30143518572334,-0.303218781300911,
-1.4614828667669));
#10729=CARTESIAN_POINT('Ctrl Pts',(1.330659040657,-0.3351607303803,-1.43511940046341));
#10730=CARTESIAN_POINT('Ctrl Pts',(1.37853719107178,-0.3732673312795,-1.38902931937536));
#10731=CARTESIAN_POINT('Ctrl Pts',(1.40296654335764,-0.387903357081022,
-1.36449833130133));
#10732=CARTESIAN_POINT('Ctrl Pts',(1.45214121543005,-0.40704475551587,-1.31204295246889));
#10733=CARTESIAN_POINT('Ctrl Pts',(1.47686834938291,-0.411552957311693,
-1.284102548491));
#10734=CARTESIAN_POINT('Ctrl Pts',(1.52104964294098,-0.411552957311693,
-1.23144933316771));
#10735=CARTESIAN_POINT('Ctrl Pts',(1.54427174765086,-0.407044755515871,
-1.20224605970712));
#10736=CARTESIAN_POINT('Ctrl Pts',(1.5873911192195,-0.387903357081022,-1.1447096804553));
#10737=CARTESIAN_POINT('Ctrl Pts',(1.60730731395783,-0.3732673312795,-1.11639170354769));
#10738=CARTESIAN_POINT('Ctrl Pts',(1.64438322958071,-0.3351607303803,-1.06123747122987));
#10739=CARTESIAN_POINT('Ctrl Pts',(1.66527150643903,-0.303218781300911,
-1.02787962443771));
#10740=CARTESIAN_POINT('Ctrl Pts',(1.69580594901181,-0.236239311587943,
-0.976785804874841));
#10741=CARTESIAN_POINT('Ctrl Pts',(1.70911544962889,-0.192537547974292,
-0.952957916220028));
#10742=CARTESIAN_POINT('Ctrl Pts',(1.72169532435455,-0.123845306465941,
-0.929898398578876));
#10743=CARTESIAN_POINT('Ctrl Pts',(1.72470909046691,-0.10165971810728,-0.924270876285509));
#10744=CARTESIAN_POINT('Ctrl Pts',(1.72679724097776,-0.0793800000000002,
-0.920353018170518));
#10745=CARTESIAN_POINT('',(1.91439494746182,-0.07938,-0.404932555664102));
#10746=CARTESIAN_POINT('Origin',(0.,-0.07938,0.));
#10747=CARTESIAN_POINT('',(1.91439494746182,-0.07938,0.404932555664102));
#10748=CARTESIAN_POINT('Ctrl Pts',(1.91439494746182,-0.0793800000000002,
-0.404932555664103));
#10749=CARTESIAN_POINT('Ctrl Pts',(1.91531368201941,-0.10165971810728,-0.400589064950645));
#10750=CARTESIAN_POINT('Ctrl Pts',(1.91662230483958,-0.123845306465941,
-0.394340921253764));
#10751=CARTESIAN_POINT('Ctrl Pts',(1.92180793393594,-0.192537547974292,
-0.368590118298695));
#10752=CARTESIAN_POINT('Ctrl Pts',(1.92692853653984,-0.236239311587943,
-0.341781714515643));
#10753=CARTESIAN_POINT('Ctrl Pts',(1.9363802706298,-0.303218781300911,-0.283014416607319));
#10754=CARTESIAN_POINT('Ctrl Pts',(1.94182093281998,-0.3351607303803,-0.244034097885537));
#10755=CARTESIAN_POINT('Ctrl Pts',(1.94887159083919,-0.3732673312795,-0.177951565523803));
#10756=CARTESIAN_POINT('Ctrl Pts',(1.95181734521941,-0.387903357081022,
-0.143456853463462));
#10757=CARTESIAN_POINT('Ctrl Pts',(1.95576966192778,-0.40704475551587,-0.071664832078622));
#10758=CARTESIAN_POINT('Ctrl Pts',(1.956752,-0.411552957311693,-0.0343669455449008));
#10759=CARTESIAN_POINT('Ctrl Pts',(1.956752,-0.411552957311693,0.0343669455449008));
#10760=CARTESIAN_POINT('Ctrl Pts',(1.95576966192778,-0.40704475551587,0.0716648320786219));
#10761=CARTESIAN_POINT('Ctrl Pts',(1.95181734521941,-0.387903357081022,
0.143456853463462));
#10762=CARTESIAN_POINT('Ctrl Pts',(1.94887159083919,-0.3732673312795,0.177951565523803));
#10763=CARTESIAN_POINT('Ctrl Pts',(1.94182093281998,-0.3351607303803,0.244034097885537));
#10764=CARTESIAN_POINT('Ctrl Pts',(1.9363802706298,-0.303218781300911,0.283014416607319));
#10765=CARTESIAN_POINT('Ctrl Pts',(1.92692853653984,-0.236239311587943,
0.341781714515643));
#10766=CARTESIAN_POINT('Ctrl Pts',(1.92180793393594,-0.192537547974292,
0.368590118298695));
#10767=CARTESIAN_POINT('Ctrl Pts',(1.91662230483958,-0.123845306465941,
0.394340921253764));
#10768=CARTESIAN_POINT('Ctrl Pts',(1.91531368201941,-0.10165971810728,0.400589064950645));
#10769=CARTESIAN_POINT('Ctrl Pts',(1.91439494746182,-0.0793800000000002,
0.404932555664103));
#10770=CARTESIAN_POINT('Origin',(0.,-0.07938,0.));
#10771=CARTESIAN_POINT('Origin',(0.,-0.07938,0.));
#10772=CARTESIAN_POINT('',(0.71358822996475,-0.07938,1.75361906569237));
#10773=CARTESIAN_POINT('Origin',(0.,-0.07938,0.));
#10774=CARTESIAN_POINT('Origin',(0.33427274200884,-0.07938,1.8957549245485));
#10775=CARTESIAN_POINT('Origin',(0.33427274200884,0.,1.8957549245485));
#10776=CARTESIAN_POINT('',(-0.070780549790825,-0.07938,1.89192444438865));
#10777=CARTESIAN_POINT('Ctrl Pts',(-0.0707805497908251,-0.07938,1.89192444438865));
#10778=CARTESIAN_POINT('Ctrl Pts',(-0.0621581887675352,-0.123392992551698,
1.89224702357808));
#10779=CARTESIAN_POINT('Ctrl Pts',(-0.0461167210878756,-0.166529565724166,
1.89282105630055));
#10780=CARTESIAN_POINT('Ctrl Pts',(-0.00546344722567869,-0.237213819614884,
1.89332631395644));
#10781=CARTESIAN_POINT('Ctrl Pts',(0.0168043156156246,-0.266247928944116,
1.89334444412923));
#10782=CARTESIAN_POINT('Ctrl Pts',(0.0676868173249578,-0.317173992396757,
1.89220877917518));
#10783=CARTESIAN_POINT('Ctrl Pts',(0.0963040116194015,-0.339063173951852,
1.89104071625784));
#10784=CARTESIAN_POINT('Ctrl Pts',(0.155686882426711,-0.373566122196588,
1.88706118493262));
#10785=CARTESIAN_POINT('Ctrl Pts',(0.189444152338378,-0.388075792674378,
1.88407517030084));
#10786=CARTESIAN_POINT('Ctrl Pts',(0.259384667806906,-0.407069005705619,
1.87572597447038));
#10787=CARTESIAN_POINT('Ctrl Pts',(0.295564880870602,-0.411552957311693,
1.87033833905209));
#10788=CARTESIAN_POINT('Ctrl Pts',(0.361953249272518,-0.411552957311693,
1.85863227849762));
#10789=CARTESIAN_POINT('Ctrl Pts',(0.397794208344885,-0.407069005705619,
1.85132063808607));
#10790=CARTESIAN_POINT('Ctrl Pts',(0.466372387779211,-0.388075792674377,
1.83524525067264));
#10791=CARTESIAN_POINT('Ctrl Pts',(0.499115122365417,-0.373566122196588,
1.82650552029421));
#10792=CARTESIAN_POINT('Ctrl Pts',(0.55627784773835,-0.339063173951852,
1.8099349185301));
#10793=CARTESIAN_POINT('Ctrl Pts',(0.583568715090836,-0.317173992396757,
1.80124488173997));
#10794=CARTESIAN_POINT('Ctrl Pts',(0.631771046764577,-0.266247928944116,
1.78490921718958));
#10795=CARTESIAN_POINT('Ctrl Pts',(0.652689698303665,-0.237213819614884,
1.77727615696148));
#10796=CARTESIAN_POINT('Ctrl Pts',(0.690718471466875,-0.166529565724165,
1.76289713151763));
#10797=CARTESIAN_POINT('Ctrl Pts',(0.705596189518013,-0.123392992551698,
1.75687121212928));
#10798=CARTESIAN_POINT('Ctrl Pts',(0.71358822996475,-0.07938,1.75361906569237));
#10799=CARTESIAN_POINT('Origin',(0.33427274200884,-0.07938,1.8957549245485));
#10800=CARTESIAN_POINT('Origin',(0.,-0.07938,0.));
#10801=CARTESIAN_POINT('',(-0.580564309297537,-0.07938,1.80203581326062));
#10802=CARTESIAN_POINT('Origin',(0.,-0.07938,0.));
#10803=CARTESIAN_POINT('Origin',(-0.962500000000001,-0.07938,1.66709890228504));
#10804=CARTESIAN_POINT('Origin',(-0.962500000000001,0.,1.66709890228504));
#10805=CARTESIAN_POINT('',(-1.27032663816428,-0.07938,1.40380134701254));
#10806=CARTESIAN_POINT('Ctrl Pts',(-1.27032663816428,-0.07938,1.40380134701254));
#10807=CARTESIAN_POINT('Ctrl Pts',(-1.26392887632193,-0.123392992551698,
1.40959080384008));
#10808=CARTESIAN_POINT('Ctrl Pts',(-1.25200938026802,-0.166529565724166,
1.42034179508297));
#10809=CARTESIAN_POINT('Ctrl Pts',(-1.22119193909219,-0.237213819614885,
1.44686026563443));
#10810=CARTESIAN_POINT('Ctrl Pts',(-1.20414549695735,-0.266247928944117,
1.46118759620237));
#10811=CARTESIAN_POINT('Ctrl Pts',(-1.16443724790971,-0.317173992396758,
1.49302426802369));
#10812=CARTESIAN_POINT('Ctrl Pts',(-1.14176438887219,-0.339063173951853,
1.51052425783311));
#10813=CARTESIAN_POINT('Ctrl Pts',(-1.09371647724559,-0.373566122196589,
1.54564633355776));
#10814=CARTESIAN_POINT('Ctrl Pts',(-1.06593753500724,-0.388075792674378,
1.56505766847808));
#10815=CARTESIAN_POINT('Ctrl Pts',(-1.00699323215303,-0.407069005705619,
1.6036187101659));
#10816=CARTESIAN_POINT('Ctrl Pts',(-0.975814475692339,-0.411552957311693,
1.62274773466534));
#10817=CARTESIAN_POINT('Ctrl Pts',(-0.917433524307661,-0.411552957311693,
1.65645399266283));
#10818=CARTESIAN_POINT('Ctrl Pts',(-0.885277924911194,-0.407069005705619,
1.67389107556648));
#10819=CARTESIAN_POINT('Ctrl Pts',(-0.822410931786043,-0.388075792674377,
1.70565781840267));
#10820=CARTESIAN_POINT('Ctrl Pts',(-0.791710751504505,-0.373566122196588,
1.72000942061118));
#10821=CARTESIAN_POINT('Ctrl Pts',(-0.737270185880016,-0.339063173951852,
1.74405909481629));
#10822=CARTESIAN_POINT('Ctrl Pts',(-0.710778320620332,-0.317173992396757,
1.75494437181449));
#10823=CARTESIAN_POINT('Ctrl Pts',(-0.663352829527299,-0.266247928944116,
1.77341438831889));
#10824=CARTESIAN_POINT('Ctrl Pts',(-0.642421776219621,-0.237213819614884,
1.78101337496783));
#10825=CARTESIAN_POINT('Ctrl Pts',(-0.604047386464641,-0.166529565724165,
1.79444282663));
#10826=CARTESIAN_POINT('Ctrl Pts',(-0.588777006905475,-0.123392992551698,
1.79938991739155));
#10827=CARTESIAN_POINT('Ctrl Pts',(-0.580564309297537,-0.0793799999999999,
1.80203581326062));
#10828=CARTESIAN_POINT('Origin',(-0.962500000000001,-0.07938,1.66709890228504));
#10829=CARTESIAN_POINT('Origin',(0.,-0.07938,0.));
#10830=CARTESIAN_POINT('',(-1.60306435598592,-0.07938,1.00725997640701));
#10831=CARTESIAN_POINT('Origin',(0.,-0.07938,0.));
#10832=CARTESIAN_POINT('Origin',(-1.80890829501287,-0.07938,0.658388775901912));
#10833=CARTESIAN_POINT('Origin',(-1.80890829501287,0.,0.658388775901912));
#10834=CARTESIAN_POINT('',(-1.8754727744327,-0.07938,0.258823997855139));
#10835=CARTESIAN_POINT('Ctrl Pts',(-1.8754727744327,-0.07938,0.258823997855138));
#10836=CARTESIAN_POINT('Ctrl Pts',(-1.87429319564052,-0.123392992551698,
0.267371381128541));
#10837=CARTESIAN_POINT('Ctrl Pts',(-1.87207293588642,-0.166529565724165,
0.283268822605344));
#10838=CARTESIAN_POINT('Ctrl Pts',(-1.86551115062085,-0.237213819614884,
0.323392218961362));
#10839=CARTESIAN_POINT('Ctrl Pts',(-1.86166224891746,-0.266247928944116,
0.34532483272118));
#10840=CARTESIAN_POINT('Ctrl Pts',(-1.85170818356893,-0.317173992396757,
0.395237108747477));
#10841=CARTESIAN_POINT('Ctrl Pts',(-1.84558854251276,-0.339063173951852,
0.423216711561106));
#10842=CARTESIAN_POINT('Ctrl Pts',(-1.83135774191,-0.373566122196588,0.481006384765672));
#10843=CARTESIAN_POINT('Ctrl Pts',(-1.82255520314685,-0.388075792674377,
0.513732289895913));
#10844=CARTESIAN_POINT('Ctrl Pts',(-1.8021878073054,-0.407069005705619,
0.581160429138046));
#10845=CARTESIAN_POINT('Ctrl Pts',(-1.79059939410895,-0.411552957311693,
0.615855430396488));
#10846=CARTESIAN_POINT('Ctrl Pts',(-1.76754295572641,-0.411552957311693,
0.679202474225583));
#10847=CARTESIAN_POINT('Ctrl Pts',(-1.75411867833313,-0.407069005705619,
0.713229275562222));
#10848=CARTESIAN_POINT('Ctrl Pts',(-1.72637903628921,-0.388075792674378,
0.777974136626975));
#10849=CARTESIAN_POINT('Ctrl Pts',(-1.71208636586057,-0.373566122196588,
0.808701797248777));
#10850=CARTESIAN_POINT('Ctrl Pts',(-1.68584130567972,-0.339063173951852,
0.862118637580169));
#10851=CARTESIAN_POINT('Ctrl Pts',(-1.67254428069212,-0.317173992396757,
0.88748588628286));
#10852=CARTESIAN_POINT('Ctrl Pts',(-1.64808654453785,-0.266247928944116,
0.932119257848273));
#10853=CARTESIAN_POINT('Ctrl Pts',(-1.63693696192699,-0.237213819614884,
0.951394641067894));
#10854=CARTESIAN_POINT('Ctrl Pts',(-1.61617275903043,-0.166529565724165,
0.986348780151617));
#10855=CARTESIAN_POINT('Ctrl Pts',(-1.60765489827034,-0.123392992551698,
0.999954082314951));
#10856=CARTESIAN_POINT('Ctrl Pts',(-1.60306435598592,-0.07938,1.00725997640701));
#10857=CARTESIAN_POINT('Origin',(-1.80890829501287,-0.07938,0.658388775901912));
#10858=CARTESIAN_POINT('Origin',(0.,-0.07938,0.));
#10859=CARTESIAN_POINT('',(-1.893248,-0.0793799999999999,2.31856010319213E-16));
#10860=CARTESIAN_POINT('Origin',(0.,-0.07938,0.));
#10861=CARTESIAN_POINT('',(-1.8754727744327,-0.07938,-0.258823997855139));
#10862=CARTESIAN_POINT('Origin',(0.,-0.07938,0.));
#10863=CARTESIAN_POINT('Origin',(-1.80890829501287,-0.07938,-0.658388775901913));
#10864=CARTESIAN_POINT('Origin',(-1.80890829501287,0.,-0.658388775901913));
#10865=CARTESIAN_POINT('',(-1.60306435598592,-0.07938,-1.00725997640701));
#10866=CARTESIAN_POINT('Ctrl Pts',(-1.60306435598592,-0.07938,-1.00725997640701));
#10867=CARTESIAN_POINT('Ctrl Pts',(-1.60765489827034,-0.123392992551698,
-0.999954082314952));
#10868=CARTESIAN_POINT('Ctrl Pts',(-1.61617275903043,-0.166529565724166,
-0.986348780151617));
#10869=CARTESIAN_POINT('Ctrl Pts',(-1.63693696192699,-0.237213819614884,
-0.951394641067894));
#10870=CARTESIAN_POINT('Ctrl Pts',(-1.64808654453785,-0.266247928944116,
-0.932119257848273));
#10871=CARTESIAN_POINT('Ctrl Pts',(-1.67254428069212,-0.317173992396757,
-0.88748588628286));
#10872=CARTESIAN_POINT('Ctrl Pts',(-1.68584130567972,-0.339063173951852,
-0.862118637580169));
#10873=CARTESIAN_POINT('Ctrl Pts',(-1.71208636586057,-0.373566122196588,
-0.808701797248777));
#10874=CARTESIAN_POINT('Ctrl Pts',(-1.72637903628921,-0.388075792674377,
-0.777974136626975));
#10875=CARTESIAN_POINT('Ctrl Pts',(-1.75411867833313,-0.407069005705619,
-0.713229275562223));
#10876=CARTESIAN_POINT('Ctrl Pts',(-1.76754295572641,-0.411552957311693,
-0.679202474225584));
#10877=CARTESIAN_POINT('Ctrl Pts',(-1.79059939410895,-0.411552957311693,
-0.615855430396488));
#10878=CARTESIAN_POINT('Ctrl Pts',(-1.8021878073054,-0.407069005705619,
-0.581160429138047));
#10879=CARTESIAN_POINT('Ctrl Pts',(-1.82255520314685,-0.388075792674378,
-0.513732289895914));
#10880=CARTESIAN_POINT('Ctrl Pts',(-1.83135774191,-0.373566122196588,-0.481006384765673));
#10881=CARTESIAN_POINT('Ctrl Pts',(-1.84558854251276,-0.339063173951852,
-0.423216711561107));
#10882=CARTESIAN_POINT('Ctrl Pts',(-1.85170818356893,-0.317173992396757,
-0.395237108747477));
#10883=CARTESIAN_POINT('Ctrl Pts',(-1.86166224891746,-0.266247928944116,
-0.34532483272118));
#10884=CARTESIAN_POINT('Ctrl Pts',(-1.86551115062085,-0.237213819614884,
-0.323392218961362));
#10885=CARTESIAN_POINT('Ctrl Pts',(-1.87207293588642,-0.166529565724166,
-0.283268822605344));
#10886=CARTESIAN_POINT('Ctrl Pts',(-1.87429319564052,-0.123392992551698,
-0.267371381128542));
#10887=CARTESIAN_POINT('Ctrl Pts',(-1.8754727744327,-0.07938,-0.258823997855139));
#10888=CARTESIAN_POINT('Origin',(-1.80890829501287,-0.07938,-0.658388775901913));
#10889=CARTESIAN_POINT('Origin',(0.,-0.07938,0.));
#10890=CARTESIAN_POINT('',(-1.27032663816428,-0.07938,-1.40380134701254));
#10891=CARTESIAN_POINT('Origin',(0.,-0.07938,0.));
#10892=CARTESIAN_POINT('Origin',(-0.9625,-0.07938,-1.66709890228504));
#10893=CARTESIAN_POINT('Origin',(-0.9625,0.,-1.66709890228504));
#10894=CARTESIAN_POINT('',(-0.580564309297535,-0.07938,-1.80203581326062));
#10895=CARTESIAN_POINT('Ctrl Pts',(-0.580564309297535,-0.07938,-1.80203581326062));
#10896=CARTESIAN_POINT('Ctrl Pts',(-0.588777006905474,-0.123392992551698,
-1.79938991739155));
#10897=CARTESIAN_POINT('Ctrl Pts',(-0.60404738646464,-0.166529565724165,
-1.79444282663));
#10898=CARTESIAN_POINT('Ctrl Pts',(-0.642421776219619,-0.237213819614884,
-1.78101337496783));
#10899=CARTESIAN_POINT('Ctrl Pts',(-0.663352829527298,-0.266247928944116,
-1.77341438831889));
#10900=CARTESIAN_POINT('Ctrl Pts',(-0.71077832062033,-0.317173992396757,
-1.75494437181449));
#10901=CARTESIAN_POINT('Ctrl Pts',(-0.737270185880015,-0.339063173951852,
-1.74405909481629));
#10902=CARTESIAN_POINT('Ctrl Pts',(-0.791710751504504,-0.373566122196588,
-1.72000942061118));
#10903=CARTESIAN_POINT('Ctrl Pts',(-0.822410931786042,-0.388075792674378,
-1.70565781840267));
#10904=CARTESIAN_POINT('Ctrl Pts',(-0.885277924911194,-0.407069005705619,
-1.67389107556648));
#10905=CARTESIAN_POINT('Ctrl Pts',(-0.917433524307661,-0.411552957311693,
-1.65645399266283));
#10906=CARTESIAN_POINT('Ctrl Pts',(-0.975814475692338,-0.411552957311693,
-1.62274773466534));
#10907=CARTESIAN_POINT('Ctrl Pts',(-1.00699323215303,-0.407069005705619,
-1.60361871016591));
#10908=CARTESIAN_POINT('Ctrl Pts',(-1.06593753500724,-0.388075792674378,
-1.56505766847808));
#10909=CARTESIAN_POINT('Ctrl Pts',(-1.09371647724559,-0.373566122196588,
-1.54564633355776));
#10910=CARTESIAN_POINT('Ctrl Pts',(-1.14176438887219,-0.339063173951852,
-1.51052425783311));
#10911=CARTESIAN_POINT('Ctrl Pts',(-1.1644372479097,-0.317173992396757,
-1.49302426802369));
#10912=CARTESIAN_POINT('Ctrl Pts',(-1.20414549695735,-0.266247928944116,
-1.46118759620237));
#10913=CARTESIAN_POINT('Ctrl Pts',(-1.22119193909219,-0.237213819614884,
-1.44686026563443));
#10914=CARTESIAN_POINT('Ctrl Pts',(-1.25200938026802,-0.166529565724166,
-1.42034179508298));
#10915=CARTESIAN_POINT('Ctrl Pts',(-1.26392887632193,-0.123392992551698,
-1.40959080384008));
#10916=CARTESIAN_POINT('Ctrl Pts',(-1.27032663816428,-0.07938,-1.40380134701254));
#10917=CARTESIAN_POINT('Origin',(-0.9625,-0.07938,-1.66709890228504));
#10918=CARTESIAN_POINT('Origin',(0.,-0.07938,0.));
#10919=CARTESIAN_POINT('',(-0.0707805497908242,-0.07938,-1.89192444438865));
#10920=CARTESIAN_POINT('Origin',(0.,-0.07938,0.));
#10921=CARTESIAN_POINT('Origin',(0.334272742008841,-0.07938,-1.8957549245485));
#10922=CARTESIAN_POINT('Origin',(0.334272742008841,0.,-1.8957549245485));
#10923=CARTESIAN_POINT('',(0.71358822996475,-0.07938,-1.75361906569237));
#10924=CARTESIAN_POINT('Ctrl Pts',(0.71358822996475,-0.07938,-1.75361906569237));
#10925=CARTESIAN_POINT('Ctrl Pts',(0.705596189518014,-0.123392992551698,
-1.75687121212928));
#10926=CARTESIAN_POINT('Ctrl Pts',(0.690718471466876,-0.166529565724166,
-1.76289713151763));
#10927=CARTESIAN_POINT('Ctrl Pts',(0.652689698303666,-0.237213819614884,
-1.77727615696148));
#10928=CARTESIAN_POINT('Ctrl Pts',(0.631771046764578,-0.266247928944116,
-1.78490921718958));
#10929=CARTESIAN_POINT('Ctrl Pts',(0.583568715090837,-0.317173992396757,
-1.80124488173997));
#10930=CARTESIAN_POINT('Ctrl Pts',(0.556277847738351,-0.339063173951852,
-1.8099349185301));
#10931=CARTESIAN_POINT('Ctrl Pts',(0.499115122365417,-0.373566122196588,
-1.8265055202942));
#10932=CARTESIAN_POINT('Ctrl Pts',(0.466372387779211,-0.388075792674378,
-1.83524525067263));
#10933=CARTESIAN_POINT('Ctrl Pts',(0.397794208344886,-0.407069005705619,
-1.85132063808607));
#10934=CARTESIAN_POINT('Ctrl Pts',(0.361953249272519,-0.411552957311693,
-1.85863227849762));
#10935=CARTESIAN_POINT('Ctrl Pts',(0.295564880870602,-0.411552957311693,
-1.87033833905209));
#10936=CARTESIAN_POINT('Ctrl Pts',(0.259384667806906,-0.407069005705619,
-1.87572597447038));
#10937=CARTESIAN_POINT('Ctrl Pts',(0.189444152338379,-0.388075792674377,
-1.88407517030084));
#10938=CARTESIAN_POINT('Ctrl Pts',(0.155686882426711,-0.373566122196588,
-1.88706118493262));
#10939=CARTESIAN_POINT('Ctrl Pts',(0.096304011619402,-0.339063173951852,
-1.89104071625784));
#10940=CARTESIAN_POINT('Ctrl Pts',(0.0676868173249583,-0.317173992396757,
-1.89220877917518));
#10941=CARTESIAN_POINT('Ctrl Pts',(0.0168043156156251,-0.266247928944116,
-1.89334444412923));
#10942=CARTESIAN_POINT('Ctrl Pts',(-0.00546344722567807,-0.237213819614884,
-1.89332631395644));
#10943=CARTESIAN_POINT('Ctrl Pts',(-0.0461167210878748,-0.166529565724165,
-1.89282105630055));
#10944=CARTESIAN_POINT('Ctrl Pts',(-0.0621581887675344,-0.123392992551698,
-1.89224702357808));
#10945=CARTESIAN_POINT('Ctrl Pts',(-0.0707805497908242,-0.07938,-1.89192444438865));
#10946=CARTESIAN_POINT('Origin',(0.334272742008841,-0.07938,-1.8957549245485));
#10947=CARTESIAN_POINT('Origin',(0.,-0.07938,0.));
#10948=CARTESIAN_POINT('',(1.16188454446795,-0.07938,-1.49479506783723));
#10949=CARTESIAN_POINT('Origin',(0.,-0.07938,0.));
#10950=CARTESIAN_POINT('Origin',(1.47463555300403,-0.07938,-1.23736614864659));
#10951=CARTESIAN_POINT('Origin',(1.47463555300403,0.,-1.23736614864659));
#10952=CARTESIAN_POINT('',(1.67384490577674,-0.07938,-0.884664467981643));
#10953=CARTESIAN_POINT('Ctrl Pts',(1.67384490577674,-0.07938,-0.884664467981643));
#10954=CARTESIAN_POINT('Ctrl Pts',(1.66981308703787,-0.123392992551698,
-0.892292941263125));
#10955=CARTESIAN_POINT('Ctrl Pts',(1.66228948011831,-0.166529565724165,
-0.906472276148934));
#10956=CARTESIAN_POINT('Ctrl Pts',(1.64240040915267,-0.237213819614884,
-0.941931672888549));
#10957=CARTESIAN_POINT('Ctrl Pts',(1.63128222892223,-0.266247928944116,
-0.961225186280958));
#10958=CARTESIAN_POINT('Ctrl Pts',(1.60485746336717,-0.317173992396757,
-1.00472289289232));
#10959=CARTESIAN_POINT('Ctrl Pts',(1.58953729406031,-0.339063173951852,
-1.02892207867768));
#10960=CARTESIAN_POINT('Ctrl Pts',(1.55639948343386,-0.373566122196588,
-1.07835938768384));
#10961=CARTESIAN_POINT('Ctrl Pts',(1.53693488395083,-0.388075792674377,
-1.10610103367386));
#10962=CARTESIAN_POINT('Ctrl Pts',(1.49473401052622,-0.407069005705619,
-1.16249669890816));
#10963=CARTESIAN_POINT('Ctrl Pts',(1.4719780748558,-0.411552957311693,-1.19113586482651));
#10964=CARTESIAN_POINT('Ctrl Pts',(1.42864614483643,-0.411552957311693,
-1.24277684810113));
#10965=CARTESIAN_POINT('Ctrl Pts',(1.40439359896051,-0.407069005705619,
-1.27016020894803));
#10966=CARTESIAN_POINT('Ctrl Pts',(1.35618281536764,-0.388075792674378,
-1.32151296077672));
#10967=CARTESIAN_POINT('Ctrl Pts',(1.33224261954459,-0.373566122196588,
-1.34549913552853));
#10968=CARTESIAN_POINT('Ctrl Pts',(1.28931069477441,-0.339063173951852,
-1.38671820696899));
#10969=CARTESIAN_POINT('Ctrl Pts',(1.26813946847809,-0.317173992396757,
-1.40600777299249));
#10970=CARTESIAN_POINT('Ctrl Pts',(1.22989120215289,-0.266247928944116,
-1.4395843844684));
#10971=CARTESIAN_POINT('Ctrl Pts',(1.21282145231718,-0.237213819614884,
-1.45388393800011));
#10972=CARTESIAN_POINT('Ctrl Pts',(1.18135446441955,-0.166529565724166,
-1.47962830891229));
#10973=CARTESIAN_POINT('Ctrl Pts',(1.16869700612251,-0.123392992551698,
-1.48949983100074));
#10974=CARTESIAN_POINT('Ctrl Pts',(1.16188454446795,-0.0793799999999999,
-1.49479506783723));
#10975=CARTESIAN_POINT('Origin',(1.47463555300403,-0.07938,-1.23736614864659));
#10976=CARTESIAN_POINT('Origin',(0.,-0.27783,0.));
#10977=CARTESIAN_POINT('',(-1.893248,-0.47628,2.31856010319213E-16));
#10978=CARTESIAN_POINT('Origin',(0.,-0.47628,0.));
#10979=CARTESIAN_POINT('',(-1.893248,-0.27783,2.31856010319213E-16));
#10980=CARTESIAN_POINT('',(1.85089094746182,-0.07938,0.39823446624808));
#10981=CARTESIAN_POINT('Origin',(0.,-0.07938,0.));
#10982=CARTESIAN_POINT('',(1.85089094746182,-0.07938,-0.39823446624808));
#10983=CARTESIAN_POINT('Ctrl Pts',(1.85089094746182,-0.07938,0.39823446624808));
#10984=CARTESIAN_POINT('Ctrl Pts',(1.8527058832274,-0.123392992551698,0.38979911355147));
#10985=CARTESIAN_POINT('Ctrl Pts',(1.85605676673266,-0.166529565724166,
0.374101031547026));
#10986=CARTESIAN_POINT('Ctrl Pts',(1.86361371531181,-0.237213819614884,
0.334153109333404));
#10987=CARTESIAN_POINT('Ctrl Pts',(1.86749832648465,-0.266247928944116,
0.312226792116516));
#10988=CARTESIAN_POINT('Ctrl Pts',(1.87521556853004,-0.317173992396757,
0.261920103790797));
#10989=CARTESIAN_POINT('Ctrl Pts',(1.87903457475221,-0.339063173951852,
0.233534836983177));
#10990=CARTESIAN_POINT('Ctrl Pts',(1.88542722875009,-0.373566122196588,
0.174363087053423));
#10991=CARTESIAN_POINT('Ctrl Pts',(1.88834846679328,-0.388075792674378,
0.140600149924591));
#10992=CARTESIAN_POINT('Ctrl Pts',(1.89227115706422,-0.407069005705619,
0.0702723654005715));
#10993=CARTESIAN_POINT('Ctrl Pts',(1.893248,-0.411552957311693,0.0337062579974903));
#10994=CARTESIAN_POINT('Ctrl Pts',(1.893248,-0.411552957311693,-0.0337062579974903));
#10995=CARTESIAN_POINT('Ctrl Pts',(1.89227115706422,-0.407069005705619,
-0.0702723654005715));
#10996=CARTESIAN_POINT('Ctrl Pts',(1.88834846679328,-0.388075792674378,
-0.140600149924591));
#10997=CARTESIAN_POINT('Ctrl Pts',(1.88542722875009,-0.373566122196588,
-0.174363087053422));
#10998=CARTESIAN_POINT('Ctrl Pts',(1.87903457475221,-0.339063173951852,
-0.233534836983177));
#10999=CARTESIAN_POINT('Ctrl Pts',(1.87521556853004,-0.317173992396757,
-0.261920103790797));
#11000=CARTESIAN_POINT('Ctrl Pts',(1.86749832648465,-0.266247928944116,
-0.312226792116516));
#11001=CARTESIAN_POINT('Ctrl Pts',(1.86361371531181,-0.237213819614884,
-0.334153109333404));
#11002=CARTESIAN_POINT('Ctrl Pts',(1.85605676673266,-0.166529565724166,
-0.374101031547026));
#11003=CARTESIAN_POINT('Ctrl Pts',(1.8527058832274,-0.123392992551698,-0.38979911355147));
#11004=CARTESIAN_POINT('Ctrl Pts',(1.85089094746182,-0.07938,-0.39823446624808));
#11005=CARTESIAN_POINT('Origin',(0.,-0.07938,0.));
#11006=CARTESIAN_POINT('Origin',(0.,-0.07938,0.));
#11007=CARTESIAN_POINT('Origin',(1.925,-0.07938,0.));
#11008=CARTESIAN_POINT('Origin',(1.925,0.,0.));
#11009=CARTESIAN_POINT('Origin',(1.925,-0.07938,0.));
#11010=CARTESIAN_POINT('Origin',(0.,-0.47628,0.));
#11011=CARTESIAN_POINT('Origin',(0.,-0.07938,0.));
#12709=UNCERTAINTY_MEASURE_WITH_UNIT(LENGTH_MEASURE(0.001),#12784,
'DISTANCE_ACCURACY_VALUE',
'Maximum model space distance between geometric entities at asserted c
onnectivities');
#12739=UNCERTAINTY_MEASURE_WITH_UNIT(LENGTH_MEASURE(0.001),#12784,
'DISTANCE_ACCURACY_VALUE',
'Maximum model space distance between geometric entities at asserted c
onnectivities');
#12753=(
GEOMETRIC_REPRESENTATION_CONTEXT(3)
GLOBAL_UNCERTAINTY_ASSIGNED_CONTEXT((#12709))
GLOBAL_UNIT_ASSIGNED_CONTEXT((#12784,#12786,#12787))
REPRESENTATION_CONTEXT('','3D')
);
#12783=(
GEOMETRIC_REPRESENTATION_CONTEXT(3)
GLOBAL_UNCERTAINTY_ASSIGNED_CONTEXT((#12739))
GLOBAL_UNIT_ASSIGNED_CONTEXT((#12784,#12786,#12787))
REPRESENTATION_CONTEXT('','3D')
);
#12784=(
LENGTH_UNIT()
NAMED_UNIT(*)
SI_UNIT(.CENTI.,.METRE.)
);
#12786=(
NAMED_UNIT(*)
PLANE_ANGLE_UNIT()
SI_UNIT($,.RADIAN.)
);
#12787=(
NAMED_UNIT(*)
SI_UNIT($,.STERADIAN.)
SOLID_ANGLE_UNIT()
);
#12801=SHAPE_DEFINITION_REPRESENTATION(#12844,#12944);
#12844=PRODUCT_DEFINITION_SHAPE('',$,#12988);
#12944=SHAPE_REPRESENTATION('',(#7217),#12753);
#12974=PRODUCT_DEFINITION_CONTEXT('part definition',#13105,'design');
#12988=PRODUCT_DEFINITION('Cage','Cage',#13031,#12974);
#13031=PRODUCT_DEFINITION_FORMATION('',$,#13120);
#13105=APPLICATION_CONTEXT(
'Core Data for Automotive Mechanical Design Process');
#13106=PRODUCT_CONTEXT('part definition',#13105,'mechanical');
#13120=PRODUCT('Cage','Cage','Cage',(#13106));
#13206=COLOUR_RGB('Grey',0.48,0.52,0.57);
#13207=FILL_AREA_STYLE_COLOUR('',#13206);
#13208=FILL_AREA_STYLE('',(#13207));
#13209=SURFACE_STYLE_FILL_AREA(#13208);
#13210=SURFACE_SIDE_STYLE('',(#13209));
#13211=SURFACE_STYLE_USAGE(.BOTH.,#13210);
#13212=PRESENTATION_STYLE_ASSIGNMENT((#13211));
ENDSEC;
END-ISO-10303-21;
